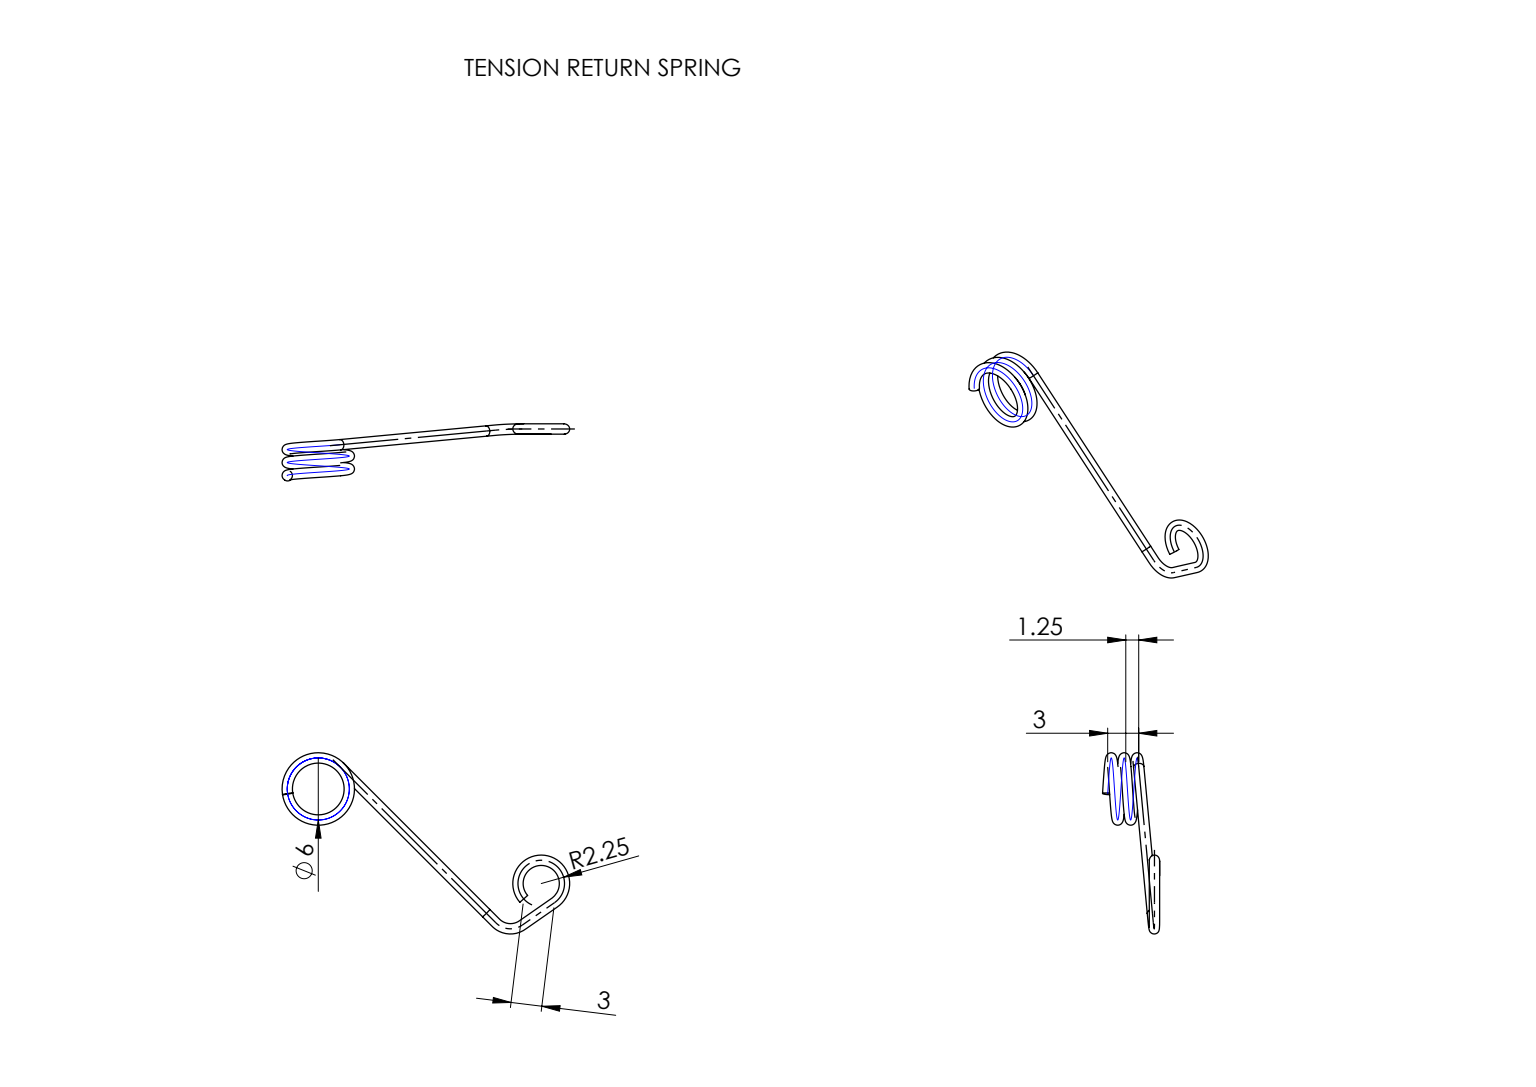
ISO-10303-21;
HEADER;
FILE_DESCRIPTION (('STEP AP214'),
    '1' );
FILE_NAME ('Tension Return Spring.step',
    '2026-10-08T05:45:04',
    ( '' ),
    ( '' ),
    'SwSTEP 2.0',
    'SolidWorks 2026',
    '' );
FILE_SCHEMA (( 'AUTOMOTIVE_DESIGN' ));
ENDSEC;

DATA;
#1=CARTESIAN_POINT ( 'NONE',  ( 16.54959645279592451, 16.98593745313911896, 13.11591282735340336 ) ) ;
#3=CARTESIAN_POINT ( 'NONE',  ( 16.03488360228399046, 17.50065030364834939, 12.16198771834506509 ) ) ;
#5=CARTESIAN_POINT ( 'NONE',  ( 22.63806431670481700, 19.48506897666907989, 12.00579112326951758 ) ) ;
#7=CARTESIAN_POINT ( 'NONE',  ( -2.527408190673963162, 30.96936468028755840, 15.39281658473306358 ) ) ;
#13=ORIENTED_EDGE ( 'NONE', *, *, #10452, .T. ) ;
#17=CARTESIAN_POINT ( 'NONE',  ( 19.95755123817951215, 17.62047157401400810, 12.00579112326941988 ) ) ;
#19=CARTESIAN_POINT ( 'NONE',  ( -2.500000000000005329, 29.80321974748362734, 16.48359592357600789 ) ) ;
#44=CARTESIAN_POINT ( 'NONE',  ( 21.41951502703731691, 22.64547864373410135, 12.00579112326941988 ) ) ;
#48=CARTESIAN_POINT ( 'NONE',  ( 22.57450250028656669, 18.29201386669844709, 10.95195840513859231 ) ) ;
#57=CARTESIAN_POINT ( 'NONE',  ( 3.472591809326047052, 31.51591669395100936, 13.67406658473306535 ) ) ;
#59=CARTESIAN_POINT ( 'NONE',  ( 18.70477062293933557, 21.09978808922912208, 12.94889058896590583 ) ) ;
#60=CARTESIAN_POINT ( 'NONE',  ( 16.65878245872646701, 16.87675144720473952, 12.10347664333366247 ) ) ;
#61=CARTESIAN_POINT ( 'NONE',  ( 17.36588923991300604, 17.58385822839129986, 12.10347664333366247 ) ) ;
#63=CARTESIAN_POINT ( 'NONE',  ( -2.500000000000003997, 29.93383077435482065, 15.47094158473306535 ) ) ;
#71=CARTESIAN_POINT ( 'NONE',  ( 19.29066956973784386, 17.16581860495888634, 12.00630190750973370 ) ) ;
#92=CARTESIAN_POINT ( 'NONE',  ( 20.23853826540680600, 19.71164639310234534, 12.00579112326941988 ) ) ;
#109=CARTESIAN_POINT ( 'NONE',  ( 16.61199375056689931, 16.92354015536430722, 11.10566822806672427 ) ) ;
#116=CARTESIAN_POINT ( 'NONE',  ( -2.521662442312484931, 32.42808502599334730, 12.81469158473306713 ) ) ;
#118=CARTESIAN_POINT ( 'NONE',  ( 22.45649315185626094, 23.58010107951569623, 12.94889058896590583 ) ) ;
#121=CARTESIAN_POINT ( 'NONE',  ( 19.90085419568980640, 16.36478119802090703, 11.95042571680015442 ) ) ;
#122=CARTESIAN_POINT ( 'NONE',  ( 19.29066956973784386, 17.16581860495888634, 12.00630190750973370 ) ) ;
#124=CARTESIAN_POINT ( 'NONE',  ( 2.500000000000008438, 30.00000000000000711, 14.59375000000000178 ) ) ;
#136=CARTESIAN_POINT ( 'NONE',  ( 23.04535143233503192, 19.92821688535955360, 12.00579112326941988 ) ) ;
#140=DIRECTION ( 'NONE',  ( 0.7512361908166118596, 0.6577071706380241967, 0.05536662621717060306 ) ) ;
#145=CARTESIAN_POINT ( 'NONE',  ( 1.101703131577913553, 32.47259180932605460, 17.07593341526694530 ) ) ;
#148=CARTESIAN_POINT ( 'NONE',  ( 2.500000000000007550, 31.03553390593274486, 14.67187500000000178 ) ) ;
#164=CARTESIAN_POINT ( 'NONE',  ( 18.88912242859132107, 19.99746927611068870, 11.95042449705224819 ) ) ;
#173=CARTESIAN_POINT ( 'NONE',  ( -1.515916693951010252, 33.47259180932604750, 13.98656658473306713 ) ) ;
#175=CARTESIAN_POINT ( 'NONE',  ( 22.08651808663882932, 17.88512374315008557, 11.95042449705224819 ) ) ;
#177=CARTESIAN_POINT ( 'NONE',  ( 23.34652552892808330, 18.77429515943753202, 11.95042449705224819 ) ) ;
#196=CARTESIAN_POINT ( 'NONE',  ( -1.814555661125937247, 28.27902175519318817, 16.37280841526694175 ) ) ;
#197=CARTESIAN_POINT ( 'NONE',  ( -2.500000000000005773, 29.99999999999999645, 13.96875000000000355 ) ) ;
#198=UNCERTAINTY_MEASURE_WITH_UNIT (LENGTH_MEASURE( 1.000000000000000082E-05 ), #3270, 'distance_accuracy_value', 'NONE');
#212=CARTESIAN_POINT ( 'NONE',  ( 24.35722724902042202, 20.98982846826517346, 11.95042449705185739 ) ) ;
#213=CARTESIAN_POINT ( 'NONE',  ( 3.500000000000007550, 28.55025253169416644, 15.76562500000000178 ) ) ;
#220=CARTESIAN_POINT ( 'NONE',  ( -0.06616922564517661864, 33.50000000000000000, 12.65844158473306535 ) ) ;
#223=CARTESIAN_POINT ( 'NONE',  ( 24.37916169550391032, 20.40431285142311424, 12.94889058896590761 ) ) ;
#226=CARTESIAN_POINT ( 'NONE',  ( 18.76105380172462844, 21.09515122317004909, 11.95042449705224819 ) ) ;
#228=FACE_OUTER_BOUND ( 'NONE', #3011, .T. ) ;
#235=CARTESIAN_POINT ( 'NONE',  ( 16.74199038346592872, 18.20775708483950694, 12.16198771834549497 ) ) ;
#244=CARTESIAN_POINT ( 'NONE',  ( 1.449747468305833120, 33.50000000000000000, 16.07812500000000355 ) ) ;
#249=CARTESIAN_POINT ( 'NONE',  ( -1.767766952966370209, 28.23223304703362402, 15.37500000000000355 ) ) ;
#250=CARTESIAN_POINT ( 'NONE',  ( -2.500000000000005773, 29.99999999999999645, 16.46875000000000355 ) ) ;
#271=CARTESIAN_POINT ( 'NONE',  ( 23.84774077504003031, 19.42364242282459230, 10.95195840513859231 ) ) ;
#272=CARTESIAN_POINT ( 'NONE',  ( 2.474873734152918558, 32.47487373415292211, 16.00000000000000355 ) ) ;
#279=CARTESIAN_POINT ( 'NONE',  ( -1.814555661125939912, 31.72097824480680117, 15.31469158473306713 ) ) ;
#283=CARTESIAN_POINT ( 'NONE',  ( 23.89484671925281845, 19.39402032390267649, 11.95042449705224819 ) ) ;
#285=CARTESIAN_POINT ( 'NONE',  ( 22.06757164964230711, 19.02077357123424406, 13.00425721518307576 ) ) ;
#300=CARTESIAN_POINT ( 'NONE',  ( -1.515916693951006478, 26.52740819067394895, 16.45093341526693820 ) ) ;
#306=CARTESIAN_POINT ( 'NONE',  ( -2.500000000000007550, 30.06616922564517580, 14.96655841526694175 ) ) ;
#308=AXIS2_PLACEMENT_3D ( 'NONE', #6956, #4296, #9565 ) ;
#310=CARTESIAN_POINT ( 'NONE',  ( 19.29066956973784386, 17.16581860495888634, 12.00630190750973370 ) ) ;
#327=CARTESIAN_POINT ( 'NONE',  ( 19.66613420429507997, 17.48520406133187066, 11.00732503135576401 ) ) ;
#333=CARTESIAN_POINT ( 'NONE',  ( -2.500000000000007550, 31.03553390593274486, 13.89062500000000355 ) ) ;
#335=CARTESIAN_POINT ( 'NONE',  ( 24.30080945327229003, 20.98731269034403368, 10.95195840513820151 ) ) ;
#337=CARTESIAN_POINT ( 'NONE',  ( 19.48730207459019326, 19.05393922246431870, 11.95042449705224996 ) ) ;
#338=CARTESIAN_POINT ( 'NONE',  ( 16.95349311633468403, 16.58206632678699677, 13.07803561935715742 ) ) ;
#343=ORIENTED_EDGE ( 'NONE', *, *, #9950, .F. ) ;
#351=CARTESIAN_POINT ( 'NONE',  ( -2.521662442312484931, 32.42808502599334730, 12.81469158473306713 ) ) ;
#354=CARTESIAN_POINT ( 'NONE',  ( 2.472591809326055046, 28.89829686842209355, 16.76343341526694175 ) ) ;
#375=CARTESIAN_POINT ( 'NONE',  ( 22.78377297911024257, 19.69285065907503807, 11.00732503135576401 ) ) ;
#382=CARTESIAN_POINT ( 'NONE',  ( -2.500000000000004441, 28.96446609406725159, 14.04687500000000355 ) ) ;
#384=CARTESIAN_POINT ( 'NONE',  ( 16.45601903647678910, 17.07951486945825792, 11.12029599681952519 ) ) ;
#387=CARTESIAN_POINT ( 'NONE',  ( 18.14679736200770677, 17.01284808935846371, 13.04404649446423115 ) ) ;
#389=AXIS2_PLACEMENT_3D ( 'NONE', #8545, #5873, #9257 ) ;
#394=CARTESIAN_POINT ( 'NONE',  ( 23.17052989764754756, 21.62756661655841839, 12.00579112326981246 ) ) ;
#402=CARTESIAN_POINT ( 'NONE',  ( -0.06616922564517119243, 26.49999999999999289, 16.52905841526693820 ) ) ;
#406=CARTESIAN_POINT ( 'NONE',  ( -3.472591809326048384, 31.51591669395100936, 14.88843341526694353 ) ) ;
#407=CARTESIAN_POINT ( 'NONE',  ( -1.515916693951006478, 26.52740819067394895, 15.20093341526694353 ) ) ;
#424=CIRCLE ( 'NONE', #2569, 0.5000000000000013323 ) ;
#425=CARTESIAN_POINT ( 'NONE',  ( 23.19605965318632457, 18.72439211931539660, 10.95195840513869179 ) ) ;
#434=CARTESIAN_POINT ( 'NONE',  ( -0.06616922564517727090, 32.50000000000000711, 15.15844158473306535 ) ) ;
#437=CARTESIAN_POINT ( 'NONE',  ( 21.34610222965416071, 23.60463303817794412, 10.95195840513859231 ) ) ;
#443=CARTESIAN_POINT ( 'NONE',  ( 19.16668011427331919, 17.04844365417888596, 13.00677669558776550 ) ) ;
#451=CARTESIAN_POINT ( 'NONE',  ( 21.51635413324704160, 18.70478684647606826, 12.00579112326941988 ) ) ;
#458=CARTESIAN_POINT ( 'NONE',  ( -3.500000000000003553, 31.44974746830583356, 16.39062500000000355 ) ) ;
#464=CARTESIAN_POINT ( 'NONE',  ( -0.06616922564517033201, 27.49999999999998934, 15.27905841526694175 ) ) ;
#481=( BOUNDED_CURVE ( )  B_SPLINE_CURVE ( 3, ( #678, #7459, #10848, #6612 ),
 .UNSPECIFIED., .F., .F. ) 
 B_SPLINE_CURVE_WITH_KNOTS ( ( 4, 4 ),
 ( 0.001563228649568143037, 0.003126104531729810565 ),
 .UNSPECIFIED. ) 
 CURVE ( )  GEOMETRIC_REPRESENTATION_ITEM ( )  RATIONAL_B_SPLINE_CURVE ( ( 1.000000000000000888, 0.3333333333333335369, 0.3333333333333327042, 1.000000000000000000 ) ) 
 REPRESENTATION_ITEM ( '' )  );
#484=AXIS2_PLACEMENT_3D ( 'NONE', #7051, #937, #5776 ) ;
#485=CARTESIAN_POINT ( 'NONE',  ( 21.34610222965416071, 23.60463303817794412, 10.95195840513859231 ) ) ;
#497=CARTESIAN_POINT ( 'NONE',  ( 16.37803167940877458, 17.15750222652490820, 11.12760988119559258 ) ) ;
#502=CARTESIAN_POINT ( 'NONE',  ( 22.73223279825284848, 19.49146071982302075, 13.00425721518307753 ) ) ;
#508=CARTESIAN_POINT ( 'NONE',  ( 21.90605485701305000, 18.97586566459109392, 12.00579112326941988 ) ) ;
#513=CARTESIAN_POINT ( 'NONE',  ( 3.527408190673962274, 28.61642175733934934, 14.76781658473306535 ) ) ;
#518=CARTESIAN_POINT ( 'NONE',  ( -3.500000000000005329, 30.06616922564516869, 16.21655841526694175 ) ) ;
#534=CARTESIAN_POINT ( 'NONE',  ( 22.29575558078030895, 19.24694448270711788, 12.00579112326941988 ) ) ;
#540=CARTESIAN_POINT ( 'NONE',  ( 1.767766952966377314, 28.23223304703363112, 15.68750000000000355 ) ) ;
#544=CARTESIAN_POINT ( 'NONE',  ( 20.23629815768686768, 16.66554095800588797, 10.95195840513859231 ) ) ;
#546=CARTESIAN_POINT ( 'NONE',  ( 22.63773560303409127, 18.20111046790825782, 12.94889058896590583 ) ) ;
#554=CARTESIAN_POINT ( 'NONE',  ( 20.47715220320264962, 17.98190999816754498, 12.00579112326941988 ) ) ;
#561=CARTESIAN_POINT ( 'NONE',  ( 1.814555661125942132, 28.27902175519319883, 13.43969158473306713 ) ) ;
#567=CARTESIAN_POINT ( 'NONE',  ( -2.479565268636987785, 29.67421718125152452, 17.49702953738633937 ) ) ;
#571=CARTESIAN_POINT ( 'NONE',  ( -1.035533905932736420, 27.49999999999998934, 14.20312500000000355 ) ) ;
#578=CARTESIAN_POINT ( 'NONE',  ( -2.474873734152920335, 32.47487373415291501, 15.06250000000000355 ) ) ;
#585=CARTESIAN_POINT ( 'NONE',  ( 19.84380896203909828, 21.37294244821887546, 12.00579112326902731 ) ) ;
#595=CARTESIAN_POINT ( 'NONE',  ( 4.553649124439118623E-15, 27.49999999999999289, 15.53125000000000355 ) ) ;
#597=CARTESIAN_POINT ( 'NONE',  ( 17.60432978939287452, 17.35624782240900288, 11.07951759511215606 ) ) ;
#598=PRESENTATION_STYLE_ASSIGNMENT (( #4897 ) ) ;
#602=CARTESIAN_POINT ( 'NONE',  ( 19.75845051886964043, 23.09045650430892849, 12.94889058896590583 ) ) ;
#610=CARTESIAN_POINT ( 'NONE',  ( -1.515916693951006478, 26.52740819067394895, 16.45093341526693820 ) ) ;
#613=CARTESIAN_POINT ( 'NONE',  ( 19.55162244606592381, 17.33808635661342024, 12.00579012602852735 ) ) ;
#619=CARTESIAN_POINT ( 'NONE',  ( -3.472591809326043499, 28.48408330604899064, 14.29906658473306358 ) ) ;
#627=CARTESIAN_POINT ( 'NONE',  ( -3.500000000000005329, 30.06616922564516869, 14.96655841526694175 ) ) ;
#640=CARTESIAN_POINT ( 'NONE',  ( 1.449747468305836673, 26.49999999999999289, 14.35937500000000533 ) ) ;
#644=CARTESIAN_POINT ( 'NONE',  ( 19.35452611835372849, 17.20101589911864437, 12.00579185514580338 ) ) ;
#657=CARTESIAN_POINT ( 'NONE',  ( 20.21677217982034946, 21.95921345637081501, 11.00732503135595941 ) ) ;
#661=CARTESIAN_POINT ( 'NONE',  ( 22.11813463801259161, 17.83967204375498383, 12.94889058896590583 ) ) ;
#669=CARTESIAN_POINT ( 'NONE',  ( -1.720978244806810498, 31.81455566112594013, 17.31030841526694175 ) ) ;
#671=CARTESIAN_POINT ( 'NONE',  ( 19.95752144772427528, 19.94857296576799754, 13.00425721518131184 ) ) ;
#677=CARTESIAN_POINT ( 'NONE',  ( -3.500000000000001332, 29.93383077435482065, 12.97094158473306358 ) ) ;
#678=CARTESIAN_POINT ( 'NONE',  ( 15.87890888817147150, 17.65662501776163040, 12.17661548709639341 ) ) ;
#692=CARTESIAN_POINT ( 'NONE',  ( -1.767766952966375094, 31.76776695296636888, 13.81250000000000355 ) ) ;
#696=CARTESIAN_POINT ( 'NONE',  ( 17.79249663040192431, 17.21067465782413919, 12.06642298039558980 ) ) ;
#704=CARTESIAN_POINT ( 'NONE',  ( -1.035533905932736420, 27.49999999999998934, 15.45312500000000178 ) ) ;
#706=CARTESIAN_POINT ( 'NONE',  ( 17.20991452582289583, 17.73983294248524700, 12.11810441208646338 ) ) ;
#710=CARTESIAN_POINT ( 'NONE',  ( 19.07396262421655919, 19.44200532275891291, 12.94889058896472811 ) ) ;
#716=SHAPE_REPRESENTATION ( 'Tension Return Spring', ( #308 ), #3340 ) ;
#717=CARTESIAN_POINT ( 'NONE',  ( 2.521662442312485819, 32.42808502599335441, 14.49780841526694175 ) ) ;
#719=CARTESIAN_POINT ( 'NONE',  ( 24.08125446323534291, 19.61299372598402613, 12.94889058896590761 ) ) ;
#725=CARTESIAN_POINT ( 'NONE',  ( -2.500000000000003997, 29.93383077435482065, 14.22094158473306535 ) ) ;
#733=CARTESIAN_POINT ( 'NONE',  ( 23.17052989764754756, 21.62756661655841839, 12.00579112326981246 ) ) ;
#742=CARTESIAN_POINT ( 'NONE',  ( 1.767766952966377314, 28.23223304703363112, 14.43750000000000178 ) ) ;
#746=CARTESIAN_POINT ( 'NONE',  ( 19.29066956973784386, 17.16581860495888634, 12.00630190750973370 ) ) ;
#757=CARTESIAN_POINT ( 'NONE',  ( 17.65010306112908722, 17.31038946799904465, 12.07741653513508417 ) ) ;
#760=CARTESIAN_POINT ( 'NONE',  ( 18.97799213218983994, 15.95698123192398477, 12.96557279687576525 ) ) ;
#769=CARTESIAN_POINT ( 'NONE',  ( 2.521662442312485819, 32.42808502599335441, 16.99780841526693820 ) ) ;
#773=CARTESIAN_POINT ( 'NONE',  ( 20.12931512496741249, 22.03068688373604900, 13.00425721518366728 ) ) ;
#775=CARTESIAN_POINT ( 'NONE',  ( 22.60611905166032898, 18.24656216730335601, 11.95042449705224819 ) ) ;
#779=CARTESIAN_POINT ( 'NONE',  ( -2.494791681227495950, 29.73705052183845154, 15.48578750830907147 ) ) ;
#789=CARTESIAN_POINT ( 'NONE',  ( 21.51635413324704160, 18.70478684647606826, 12.00579112326941988 ) ) ;
#807=CARTESIAN_POINT ( 'NONE',  ( 19.85760542366876535, 20.31250532737884384, 12.00579112326941988 ) ) ;
#818=CARTESIAN_POINT ( 'NONE',  ( 19.66613420429507997, 17.48520406133187066, 11.00732503135576401 ) ) ;
#824=CARTESIAN_POINT ( 'NONE',  ( 15.36174878203077476, 18.17378512388119915, 11.22291988893967840 ) ) ;
#835=CARTESIAN_POINT ( 'NONE',  ( 1.383578242660657098, 33.52740819067396671, 15.08031658473306891 ) ) ;
#837=CARTESIAN_POINT ( 'NONE',  ( 19.53332707643461319, 16.11782042516817981, 12.95310296989756260 ) ) ;
#839=EDGE_CURVE ( 'NONE', #8937, #5318, #2844, .T. ) ;
#845=CARTESIAN_POINT ( 'NONE',  ( 1.035533905932737975, 32.50000000000000711, 13.57812500000000178 ) ) ;
#856=CARTESIAN_POINT ( 'NONE',  ( 22.69616945897178084, 19.53356342368596898, 12.00579112326941988 ) ) ;
#857=CARTESIAN_POINT ( 'NONE',  ( -1.035533905932736420, 27.49999999999998934, 15.45312500000000178 ) ) ;
#882=CARTESIAN_POINT ( 'NONE',  ( 22.05490153526506703, 17.93057544254518376, 10.95195840513859231 ) ) ;
#883=CARTESIAN_POINT ( 'NONE',  ( -3.456897879362374582, 29.45240795142739998, 16.49922112211940117 ) ) ;
#890=CARTESIAN_POINT ( 'NONE',  ( -3.500000000000003553, 31.44974746830583356, 16.39062500000000355 ) ) ;
#893=CARTESIAN_POINT ( 'NONE',  ( 21.85833415550051484, 17.65895283167741425, 12.94889058896590583 ) ) ;
#896=CARTESIAN_POINT ( 'NONE',  ( 17.59356678224322934, 17.35619608210146581, 12.08212522340233264 ) ) ;
#898=CARTESIAN_POINT ( 'NONE',  ( -1.767766952966370209, 28.23223304703362402, 15.37500000000000355 ) ) ;
#909=CARTESIAN_POINT ( 'NONE',  ( -2.385244779468109755E-15, 32.50000000000000711, 16.15625000000000355 ) ) ;
#937=DIRECTION ( 'NONE',  ( -0.1561119869139967753, 0.9855205127846311530, -0.06616922564517428718 ) ) ;
#939=CARTESIAN_POINT ( 'NONE',  ( 24.09141472773967507, 22.06251279622207306, 11.95042449705264076 ) ) ;
#946=CARTESIAN_POINT ( 'NONE',  ( 0.06616922564517879746, 26.50000000000000000, 13.28344158473306713 ) ) ;
#948=CARTESIAN_POINT ( 'NONE',  ( 21.34179237787287065, 23.66094220255952152, 11.95042449705224819 ) ) ;
#950=CARTESIAN_POINT ( 'NONE',  ( 18.94130700685887447, 16.00034706198404066, 11.96718634320919250 ) ) ;
#951=CARTESIAN_POINT ( 'NONE',  ( 15.88045857259785087, 19.06928889570832197, 12.24278471274156388 ) ) ;
#960=CARTESIAN_POINT ( 'NONE',  ( 18.10462311893278553, 17.05669763433401087, 12.04589798090090902 ) ) ;
#971=EDGE_LOOP ( 'NONE', ( #10177, #7485, #4128, #4625 ) ) ;
#974=CARTESIAN_POINT ( 'NONE',  ( -1.101703131577911776, 27.52740819067395250, 16.45093341526693820 ) ) ;
#994=CARTESIAN_POINT ( 'NONE',  ( 17.22114890795359798, 16.40384437412513208, 11.05348780010051435 ) ) ;
#1002=CARTESIAN_POINT ( 'NONE',  ( 1.449747468305836673, 26.49999999999999289, 15.60937500000000711 ) ) ;
#1004=CARTESIAN_POINT ( 'NONE',  ( 19.79393261808261428, 23.04652112618272852, 11.95042449705224819 ) ) ;
#1006=CARTESIAN_POINT ( 'NONE',  ( 24.35722724902042202, 20.98982846826517346, 11.95042449705185739 ) ) ;
#1007=CARTESIAN_POINT ( 'NONE',  ( 19.35452611835372849, 17.20101589911864437, 12.00579185514580338 ) ) ;
#1009=CARTESIAN_POINT ( 'NONE',  ( -2.500000000000004885, 29.80321974748363090, 16.48359592357600434 ) ) ;
#1011=CARTESIAN_POINT ( 'NONE',  ( -0.06616922564517661864, 33.50000000000000000, 15.15844158473306535 ) ) ;
#1021=CARTESIAN_POINT ( 'NONE',  ( -2.500000000000007550, 31.03553390593274131, 16.39062500000000355 ) ) ;
#1030=CARTESIAN_POINT ( 'NONE',  ( -2.500000000000005773, 29.99999999999999645, 15.21875000000000355 ) ) ;
#1032=CARTESIAN_POINT ( 'NONE',  ( 1.767766952966372429, 31.76776695296637598, 14.75000000000000355 ) ) ;
#1048=CARTESIAN_POINT ( 'NONE',  ( 19.86895450806392560, 16.41003605044161162, 10.95195963068177392 ) ) ;
#1049=CARTESIAN_POINT ( 'NONE',  ( -2.474873734152920335, 32.47487373415291501, 16.31250000000000355 ) ) ;
#1051=ADVANCED_FACE ( 'NONE', ( #228 ), #4624, .T. ) ;
#1056=CARTESIAN_POINT ( 'NONE',  ( -2.521662442312484931, 32.42808502599334730, 14.06469158473306358 ) ) ;
#1058=CARTESIAN_POINT ( 'NONE',  ( 23.34652552892808330, 18.77429515943753202, 11.95042449705224819 ) ) ;
#1060=CARTESIAN_POINT ( 'NONE',  ( 23.64018263364375017, 19.06693133664117212, 11.95042449705224819 ) ) ;
#1061=CARTESIAN_POINT ( 'NONE',  ( 22.45328846257175925, 22.40877220821986171, 12.00579112326941988 ) ) ;
#1077=CARTESIAN_POINT ( 'NONE',  ( -3.472591809326048384, 31.51591669395100936, 17.38843341526693820 ) ) ;
#1082=CARTESIAN_POINT ( 'NONE',  ( 2.500000000000010214, 28.96446609406726225, 14.51562500000000355 ) ) ;
#1102=CARTESIAN_POINT ( 'NONE',  ( 21.87443830563928415, 19.02131736398618855, 11.00732503135576401 ) ) ;
#1110=CARTESIAN_POINT ( 'NONE',  ( -2.500000000000003997, 29.93383077435482065, 12.97094158473306358 ) ) ;
#1113=CARTESIAN_POINT ( 'NONE',  ( 20.26791470906062997, 16.62008925861079334, 11.95042449705224819 ) ) ;
#1116=CARTESIAN_POINT ( 'NONE',  ( 19.79393261808261428, 23.04652112618272852, 11.95042449705224819 ) ) ;
#1118=CARTESIAN_POINT ( 'NONE',  ( 19.05040816462259556, 17.06282649731835122, 12.00984920396035172 ) ) ;
#1124=CARTESIAN_POINT ( 'NONE',  ( 17.45361707773674809, 17.49611573659335662, 12.09524845743996657 ) ) ;
#1131=CARTESIAN_POINT ( 'NONE',  ( -1.734723475976807094E-15, 33.50000000000000000, 16.15625000000000355 ) ) ;
#1136=CARTESIAN_POINT ( 'NONE',  ( -2.385244779468109755E-15, 32.50000000000000711, 14.90625000000000355 ) ) ;
#1137=CARTESIAN_POINT ( 'NONE',  ( -3.456897879362374582, 29.45240795142739998, 16.49922112211940117 ) ) ;
#1159=CARTESIAN_POINT ( 'NONE',  ( 24.30080945327229003, 20.98731269034403368, 10.95195840513820151 ) ) ;
#1166=CARTESIAN_POINT ( 'NONE',  ( 2.472591809326049272, 31.10170313157791711, 14.92406658473306713 ) ) ;
#1169=CARTESIAN_POINT ( 'NONE',  ( 24.41364504476855402, 20.99234424618630257, 12.94889058896551326 ) ) ;
#1170=APPLICATION_CONTEXT ( 'automotive_design' ) ;
#1172=CARTESIAN_POINT ( 'NONE',  ( 17.41267794807257374, 17.53706952023173216, 13.10128505860060066 ) ) ;
#1175=SURFACE_SIDE_STYLE ('',( #8791 ) ) ;
#1182=CARTESIAN_POINT ( 'NONE',  ( 17.20991452582289583, 17.73983294248524700, 12.11810441208646338 ) ) ;
#1190=CARTESIAN_POINT ( 'NONE',  ( 2.474873734152922111, 27.52512626584708144, 15.68750000000000355 ) ) ;
#1194=ADVANCED_FACE ( 'NONE', ( #10156 ), #7826, .T. ) ;
#1195=CARTESIAN_POINT ( 'NONE',  ( 0.06616922564517249694, 32.50000000000000711, 15.90405841526694175 ) ) ;
#1198=CARTESIAN_POINT ( 'NONE',  ( -2.500000000000005773, 29.99999999999999645, 15.21875000000000355 ) ) ;
#1222=CARTESIAN_POINT ( 'NONE',  ( 22.00433854689477897, 19.11167697002443333, 11.00732503135576401 ) ) ;
#1229=CARTESIAN_POINT ( 'NONE',  ( 1.101703131577918438, 27.52740819067395606, 13.36156658473306535 ) ) ;
#1230=ORIENTED_EDGE ( 'NONE', *, *, #839, .F. ) ;
#1231=CARTESIAN_POINT ( 'NONE',  ( 18.81733698050991777, 21.09051435711097966, 10.95195840513859231 ) ) ;
#1233=CARTESIAN_POINT ( 'NONE',  ( 22.98142095123195716, 18.50759888342988546, 11.95042449705211141 ) ) ;
#1234=CARTESIAN_POINT ( 'NONE',  ( 19.08509339279509831, 17.01892842213374735, 13.00828316275149099 ) ) ;
#1238=B_SPLINE_CURVE_WITH_KNOTS ( 'NONE', 3,
 ( #9810, #2255, #5649, #4814, #1472, #4083, #4023, #7411, #10804, #9128, #10026, #2415, #5802, #6798, #7585, #5092, #7642, #71, #4980, #6077, #10307, #17, #9361, #4257, #3418, #10253, #789, #10193, #1759, #1694, #8472, #2590, #856, #3536, #2702, #136, #5971, #5913, #10975, #733, #9296, #3364, #6918, #8579, #6743, #1581, #5150, #2475, #4196, #3306, #8354, #10139 ),
 .UNSPECIFIED., .F., .F.,
 ( 4, 2, 2, 2, 2, 2, 2, 2, 2, 2, 2, 2, 2, 2, 2, 2, 2, 2, 2, 2, 2, 2, 2, 2, 2, 4 ),
 ( 0.05059550242215297977, 0.08415034466753114339, 0.1009277657902202252, 0.1177051869129092931, 0.1353321994545625961, 0.1529592119962158714, 0.1882132370795224774, 0.2234672621628290834, 0.2410942747044824142, 0.2587212872461356894, 0.2827395206008344042, 0.3067577539555331190, 0.3547942206649305485, 0.4028306873743279781, 0.4268489207290267484, 0.4508671540837254077, 0.4680275555186089731, 0.4851879569534925385, 0.5195087598232597248, 0.5881503655627940974, 0.6567919713023284700, 0.7254335770418627316, 0.7940751827813969932, 0.8627167885209312548, 0.9313583942604657384, 1.000000000000000000 ),
 .UNSPECIFIED. ) ;
#1243=CARTESIAN_POINT ( 'NONE',  ( 15.92724728075741680, 19.02250018754875072, 13.24059312800850030 ) ) ;
#1252=CARTESIAN_POINT ( 'NONE',  ( -2.474873734152920335, 32.47487373415291501, 13.81250000000000355 ) ) ;
#1257=CARTESIAN_POINT ( 'NONE',  ( -1.383578242660661983, 33.52740819067396671, 15.98218341526694175 ) ) ;
#1258=CARTESIAN_POINT ( 'NONE',  ( 1.515916693951008254, 33.47259180932604750, 15.82593341526694353 ) ) ;
#1259=CARTESIAN_POINT ( 'NONE',  ( 22.45328846257175925, 22.40877220821986171, 12.00579112326941988 ) ) ;
#1278=CARTESIAN_POINT ( 'NONE',  ( 19.52895938645546536, 19.09041019265748673, 10.95195840513859586 ) ) ;
#1284=CARTESIAN_POINT ( 'NONE',  ( 2.472591809326049272, 31.10170313157791711, 13.67406658473306535 ) ) ;
#1286=CARTESIAN_POINT ( 'NONE',  ( 15.12656308325174415, 18.40897082268132934, 11.24497629747462568 ) ) ;
#1291=CARTESIAN_POINT ( 'NONE',  ( 17.50063742165245984, 17.44909550871243198, 13.09303515564029397 ) ) ;
#1297=CARTESIAN_POINT ( 'NONE',  ( 20.00651627240589647, 19.97666299463432438, 12.00579112326824216 ) ) ;
#1304=CARTESIAN_POINT ( 'NONE',  ( -1.383578242660661983, 33.52740819067396671, 17.23218341526694530 ) ) ;
#1308=CARTESIAN_POINT ( 'NONE',  ( 0.9693646802875698354, 27.47259180932603684, 16.60718341526694175 ) ) ;
#1328=CARTESIAN_POINT ( 'NONE',  ( 23.59820535295391508, 19.10314065948846718, 10.95195840513859231 ) ) ;
#1335=CARTESIAN_POINT ( 'NONE',  ( -2.500000000000007550, 31.03553390593274486, 15.14062500000000355 ) ) ;
#1339=CARTESIAN_POINT ( 'NONE',  ( 16.69520167530635746, 18.25454579299907465, 11.16417930307855677 ) ) ;
#1344=CARTESIAN_POINT ( 'NONE',  ( 17.25670323398246353, 17.69304423432567930, 13.11591282735340336 ) ) ;
#1353=CARTESIAN_POINT ( 'NONE',  ( 22.03595509826854126, 19.06622527062933870, 12.00579112326941988 ) ) ;
#1360=CARTESIAN_POINT ( 'NONE',  ( -3.472591809326043499, 28.48408330604899064, 13.04906658473306891 ) ) ;
#1365=CARTESIAN_POINT ( 'NONE',  ( -1.383578242660661983, 33.52740819067396671, 15.98218341526694175 ) ) ;
#1369=CARTESIAN_POINT ( 'NONE',  ( -1.035533905932742860, 32.50000000000000000, 13.73437500000000888 ) ) ;
#1374=ORIENTED_EDGE ( 'NONE', *, *, #8914, .F. ) ;
#1385=CARTESIAN_POINT ( 'NONE',  ( 18.79784185921769790, 16.99560944861731215, 12.01584860934582366 ) ) ;
#1399=CARTESIAN_POINT ( 'NONE',  ( 19.42818427286271898, 22.60367925258928068, 10.95195840513898489 ) ) ;
#1401=CARTESIAN_POINT ( 'NONE',  ( 23.09245737654782360, 19.89859478643763069, 13.00425721518307753 ) ) ;
#1409=CARTESIAN_POINT ( 'NONE',  ( 19.16668011427331919, 17.04844365417888596, 13.00677669558776550 ) ) ;
#1414=CARTESIAN_POINT ( 'NONE',  ( -3.446545381698513655, 29.38705359262400663, 15.50141270685246830 ) ) ;
#1420=CARTESIAN_POINT ( 'NONE',  ( -2.527408190673963162, 29.03063531971243094, 16.29468341526694530 ) ) ;
#1429=CARTESIAN_POINT ( 'NONE',  ( -3.500000000000003109, 29.99999999999999645, 13.96875000000000355 ) ) ;
#1434=CARTESIAN_POINT ( 'NONE',  ( 16.11564427137601285, 18.83410319690818824, 12.22072830420661660 ) ) ;
#1442=CARTESIAN_POINT ( 'NONE',  ( -2.500000000000007550, 31.03553390593274486, 16.39062500000000355 ) ) ;
#1446=CARTESIAN_POINT ( 'NONE',  ( 21.07346791105437589, 22.52558620363005915, 11.00732503135576401 ) ) ;
#1450=CARTESIAN_POINT ( 'NONE',  ( 23.83741617020655212, 22.59052263540754524, 12.94889058896590583 ) ) ;
#1455=CARTESIAN_POINT ( 'NONE',  ( 2.428085025993357071, 27.47833755768751374, 15.43530841526694175 ) ) ;
#1457=CARTESIAN_POINT ( 'NONE',  ( 20.76856923708738734, 18.11717751085002703, 13.00425721518307576 ) ) ;
#1465=CARTESIAN_POINT ( 'NONE',  ( 2.527408190673965382, 29.03063531971243449, 13.51781658473306713 ) ) ;
#1470=CARTESIAN_POINT ( 'NONE',  ( -0.06616922564517033201, 27.49999999999998934, 16.52905841526693820 ) ) ;
#1472=CARTESIAN_POINT ( 'NONE',  ( 17.20991452582289583, 17.73983294248524700, 12.11810441208646338 ) ) ;
#1479=CARTESIAN_POINT ( 'NONE',  ( -1.449747468305830678, 26.49999999999999289, 15.45312500000000178 ) ) ;
#1483=CARTESIAN_POINT ( 'NONE',  ( 19.55162244606592381, 17.33808635661342024, 12.00579012602852735 ) ) ;
#1494=CARTESIAN_POINT ( 'NONE',  ( 16.74199038346592872, 18.20775708483950694, 12.16198771834549497 ) ) ;
#1500=CARTESIAN_POINT ( 'NONE',  ( 23.58716357997163016, 18.92604383881832675, 12.94889058896590583 ) ) ;
#1506=CARTESIAN_POINT ( 'NONE',  ( -0.06616922564517119243, 26.49999999999999289, 15.27905841526694175 ) ) ;
#1509=CARTESIAN_POINT ( 'NONE',  ( 16.23764702455707720, 17.29788688137487185, 13.14516836485838169 ) ) ;
#1515=CARTESIAN_POINT ( 'NONE',  ( 1.720978244806805169, 31.81455566112594013, 12.50219158473306358 ) ) ;
#1535=CARTESIAN_POINT ( 'NONE',  ( 3.903127820947815962E-15, 26.49999999999999289, 15.53125000000000355 ) ) ;
#1540=CARTESIAN_POINT ( 'NONE',  ( 17.20991452582289583, 17.73983294248524700, 12.11810441208646338 ) ) ;
#1553=CARTESIAN_POINT ( 'NONE',  ( 22.41005638895160601, 19.39388128063383476, 11.00732503135576401 ) ) ;
#1557=CARTESIAN_POINT ( 'NONE',  ( 24.37916169550391032, 20.40431285142311424, 12.94889058896590761 ) ) ;
#1565=CARTESIAN_POINT ( 'NONE',  ( -0.06616922564517119243, 26.49999999999999289, 16.52905841526693820 ) ) ;
#1567=CARTESIAN_POINT ( 'NONE',  ( 23.18216631463591781, 20.05868775325893338, 13.00425721518307753 ) ) ;
#1573=CARTESIAN_POINT ( 'NONE',  ( -0.06616922564517727090, 32.50000000000000711, 13.90844158473306713 ) ) ;
#1581=CARTESIAN_POINT ( 'NONE',  ( 20.43380676890320657, 22.25420293214091316, 12.00579112326941988 ) ) ;
#1591=CARTESIAN_POINT ( 'NONE',  ( -2.500000000000004441, 28.96446609406725159, 14.04687500000000355 ) ) ;
#1596=CARTESIAN_POINT ( 'NONE',  ( 18.10462311893278553, 17.05669763433401087, 12.04589798090090902 ) ) ;
#1606=CARTESIAN_POINT ( 'NONE',  ( -2.500000000000004885, 29.80321974748363090, 16.48359592357600434 ) ) ;
#1608=CARTESIAN_POINT ( 'NONE',  ( 19.25788680476432546, 17.21053220311310739, 11.00783986014182148 ) ) ;
#1612=CARTESIAN_POINT ( 'NONE',  ( 24.41364504476855402, 20.99234424618630257, 12.94889058896551326 ) ) ;
#1620=CARTESIAN_POINT ( 'NONE',  ( -1.383578242660661983, 33.52740819067396671, 17.23218341526694530 ) ) ;
#1623=CARTESIAN_POINT ( 'NONE',  ( 22.50783536177859645, 18.11075086187001659, 12.94889058896590583 ) ) ;
#1625=VECTOR ( 'NONE', #10324, 999.9999999999998863 ) ;
#1626=CARTESIAN_POINT ( 'NONE',  ( 22.47621881040483771, 18.15620256126511478, 11.95042449705224819 ) ) ;
#1630=CARTESIAN_POINT ( 'NONE',  ( 1.814555661125942132, 28.27902175519319883, 14.68969158473306535 ) ) ;
#1663=CARTESIAN_POINT ( 'NONE',  ( 22.00433854689477897, 19.11167697002443333, 11.00732503135576401 ) ) ;
#1667=CARTESIAN_POINT ( 'NONE',  ( 22.43871220627207563, 23.52649944903870249, 11.95042449705224819 ) ) ;
#1674=CARTESIAN_POINT ( 'NONE',  ( 3.527408190673962274, 28.61642175733934934, 14.76781658473306535 ) ) ;
#1676=CARTESIAN_POINT ( 'NONE',  ( 23.01143949934618504, 18.46103507366711227, 12.94889058896576906 ) ) ;
#1683=CARTESIAN_POINT ( 'NONE',  ( 2.472591809326049272, 31.10170313157791711, 14.92406658473306713 ) ) ;
#1689=ADVANCED_FACE ( 'NONE', ( #4201 ), #10919, .T. ) ;
#1694=CARTESIAN_POINT ( 'NONE',  ( 22.29575558078030895, 19.24694448270711788, 12.00579112326941988 ) ) ;
#1696=CARTESIAN_POINT ( 'NONE',  ( 2.500000000000008438, 30.00000000000000711, 15.84375000000000355 ) ) ;
#1720=CARTESIAN_POINT ( 'NONE',  ( 21.25655365073496839, 18.52406763439849513, 12.00579112326941988 ) ) ;
#1726=CARTESIAN_POINT ( 'NONE',  ( 21.01569960522067504, 17.20769859423666048, 10.95195840513859231 ) ) ;
#1737=CARTESIAN_POINT ( 'NONE',  ( -3.446545381698513655, 29.38705359262400663, 15.50141270685246830 ) ) ;
#1739=CARTESIAN_POINT ( 'NONE',  ( 20.19688095354152324, 19.67517542290917731, 13.00425721518307753 ) ) ;
#1744=CARTESIAN_POINT ( 'NONE',  ( 21.05771646464872404, 22.57981893131178452, 12.00579112326941988 ) ) ;
#1746=CARTESIAN_POINT ( 'NONE',  ( -1.767766952966375094, 31.76776695296636888, 16.31250000000000355 ) ) ;
#1759=CARTESIAN_POINT ( 'NONE',  ( 22.03595509826854126, 19.06622527062933870, 12.00579112326941988 ) ) ;
#1760=CARTESIAN_POINT ( 'NONE',  ( 2.500000000000008438, 30.00000000000000711, 14.59375000000000178 ) ) ;
#1781=CARTESIAN_POINT ( 'NONE',  ( 20.08745147943499987, 17.71083118005251933, 12.00579112326941988 ) ) ;
#1786=CARTESIAN_POINT ( 'NONE',  ( 19.38445574543743177, 22.63941596627307362, 11.95042449705263898 ) ) ;
#1787=CARTESIAN_POINT ( 'NONE',  ( 3.500000000000005329, 30.00000000000000000, 15.84375000000000355 ) ) ;
#1793=CARTESIAN_POINT ( 'NONE',  ( -3.472591809326043499, 28.48408330604899064, 13.04906658473306891 ) ) ;
#1795=CARTESIAN_POINT ( 'NONE',  ( 16.72700999897183038, 16.80849948458634557, 12.09707671258119888 ) ) ;
#1798=CARTESIAN_POINT ( 'NONE',  ( 17.78598590678423719, 16.10215687441832699, 12.01726674494117653 ) ) ;
#1799=CARTESIAN_POINT ( 'NONE',  ( 20.23853826540680600, 19.71164639310234534, 12.00579112326941988 ) ) ;
#1801=CARTESIAN_POINT ( 'NONE',  ( -2.469212770973128190, 29.60886282244813117, 16.49922112211940117 ) ) ;
#1806=ORIENTED_EDGE ( 'NONE', *, *, #6807, .F. ) ;
#1818=CARTESIAN_POINT ( 'NONE',  ( -1.767766952966375094, 31.76776695296636888, 16.31250000000000355 ) ) ;
#1836=CARTESIAN_POINT ( 'NONE',  ( 20.26791470906062997, 16.62008925861079334, 11.95042449705224819 ) ) ;
#1843=CARTESIAN_POINT ( 'NONE',  ( 3.500000000000003997, 30.06616922564517580, 14.84594158473306713 ) ) ;
#1845=CARTESIAN_POINT ( 'NONE',  ( 19.76265562249496099, 16.28401831655332543, 11.95127577209155234 ) ) ;
#1850=CARTESIAN_POINT ( 'NONE',  ( 1.035533905932743970, 27.49999999999999289, 15.60937500000000711 ) ) ;
#1860=CARTESIAN_POINT ( 'NONE',  ( -2.469212770973128190, 29.60886282244813827, 16.49922112211940117 ) ) ;
#1871=CARTESIAN_POINT ( 'NONE',  ( 2.500000000000009770, 29.93383077435482420, 16.84155841526694175 ) ) ;
#1897=CARTESIAN_POINT ( 'NONE',  ( 18.60991190964745456, 16.01828113007465504, 10.97873183052796620 ) ) ;
#1906=CARTESIAN_POINT ( 'NONE',  ( -1.734723475976807094E-15, 33.50000000000000000, 16.15625000000000355 ) ) ;
#1908=CARTESIAN_POINT ( 'NONE',  ( 18.07012887690021330, 16.02595819568259827, 12.00212024154935975 ) ) ;
#1931=ORIENTED_EDGE ( 'NONE', *, *, #7024, .F. ) ;
#1934=CARTESIAN_POINT ( 'NONE',  ( 2.500000000000010214, 28.96446609406726225, 15.76562500000000178 ) ) ;
#1955=CARTESIAN_POINT ( 'NONE',  ( 16.69520167530635746, 18.25454579299907465, 11.16417930307855677 ) ) ;
#1962=CARTESIAN_POINT ( 'NONE',  ( -0.9693646802875608426, 27.47259180932603684, 14.45531658473306535 ) ) ;
#1964=CARTESIAN_POINT ( 'NONE',  ( 16.90694777372845437, 16.62861179130368683, 12.08020438729360180 ) ) ;
#1966=CARTESIAN_POINT ( 'NONE',  ( 19.95755123817951215, 17.62047157401400810, 12.00579112326941988 ) ) ;
#1979=CARTESIAN_POINT ( 'NONE',  ( -3.500000000000005329, 30.06616922564516869, 17.46655841526694175 ) ) ;
#1984=CARTESIAN_POINT ( 'NONE',  ( -2.469212770973128190, 29.60886282244813117, 16.49922112211940117 ) ) ;
#1985=CARTESIAN_POINT ( 'NONE',  ( 1.767766952966377314, 28.23223304703363112, 14.43750000000000178 ) ) ;
#2000=CARTESIAN_POINT ( 'NONE',  ( 23.26254143866440671, 20.58647472722595850, 11.00732503135576401 ) ) ;
#2002=CARTESIAN_POINT ( 'NONE',  ( -3.500000000000002665, 29.72450764647708255, 16.48359592357600789 ) ) ;
#2010=CARTESIAN_POINT ( 'NONE',  ( -1.814555661125939912, 31.72097824480680117, 14.06469158473306358 ) ) ;
#2012=CARTESIAN_POINT ( 'NONE',  ( 15.40853749019034069, 18.12699641572163145, 12.22072830420661660 ) ) ;
#2013=CARTESIAN_POINT ( 'NONE',  ( 18.86745781575159242, 21.66267592685425569, 11.95042449705185561 ) ) ;
#2014=CARTESIAN_POINT ( 'NONE',  ( 21.93767140838681584, 18.93041396519599928, 13.00425721518307576 ) ) ;
#2028=CARTESIAN_POINT ( 'NONE',  ( 3.500000000000005773, 31.44974746830583356, 14.67187500000000178 ) ) ;
#2034=CARTESIAN_POINT ( 'NONE',  ( 1.767766952966372429, 31.76776695296637598, 16.00000000000000355 ) ) ;
#2037=CARTESIAN_POINT ( 'NONE',  ( 21.51635413324704160, 18.70478684647606826, 12.00579112326941988 ) ) ;
#2057=CARTESIAN_POINT ( 'NONE',  ( 19.42818427286271898, 22.60367925258928068, 10.95195840513898489 ) ) ;
#2064=CARTESIAN_POINT ( 'NONE',  ( -2.458860273309268152, 29.54350846364475203, 15.50141270685246830 ) ) ;
#2067=CARTESIAN_POINT ( 'NONE',  ( 18.88912242859132107, 19.99746927611068870, 11.95042449705224819 ) ) ;
#2071=CARTESIAN_POINT ( 'NONE',  ( 22.92515349615029407, 19.68371071013345741, 13.00425721518307753 ) ) ;
#2079=CARTESIAN_POINT ( 'NONE',  ( 19.38642580597931087, 17.15576104669793267, 13.00425794126423362 ) ) ;
#2091=CARTESIAN_POINT ( 'NONE',  ( -1.449747468305836229, 33.50000000000000000, 14.98437500000000711 ) ) ;
#2094=CARTESIAN_POINT ( 'NONE',  ( 1.449747468305833120, 33.50000000000000000, 14.82812500000000178 ) ) ;
#2097=CARTESIAN_POINT ( 'NONE',  ( -1.035533905932742638, 32.50000000000000000, 16.23437500000000355 ) ) ;
#2105=MECHANICAL_DESIGN_GEOMETRIC_PRESENTATION_REPRESENTATION('',(#6704),#8842);
#2118=CARTESIAN_POINT ( 'NONE',  ( 22.83430298279833437, 18.47273307877622983, 10.95195840513859231 ) ) ;
#2124=CARTESIAN_POINT ( 'NONE',  ( 2.500000000000007550, 31.03553390593274486, 14.67187500000000178 ) ) ;
#2126=ORIENTED_EDGE ( 'NONE', *, *, #6854, .T. ) ;
#2128=CARTESIAN_POINT ( 'NONE',  ( 23.59820535295391508, 19.10314065948846718, 10.95195840513859231 ) ) ;
#2130=CARTESIAN_POINT ( 'NONE',  ( 19.58285320134683261, 17.29236643726018130, 13.00425622583864715 ) ) ;
#2135=CARTESIAN_POINT ( 'NONE',  ( 16.16243297953557700, 18.78731448874862053, 13.21853671947355302 ) ) ;
#2142=CARTESIAN_POINT ( 'NONE',  ( -3.500000000000003109, 29.99999999999999645, 15.21875000000000355 ) ) ;
#2148=CARTESIAN_POINT ( 'NONE',  ( -3.467250377026234176, 29.51776231023078623, 17.49702953738633937 ) ) ;
#2149=CARTESIAN_POINT ( 'NONE',  ( 0.06616922564517314920, 33.50000000000000000, 14.65405841526694353 ) ) ;
#2164=CARTESIAN_POINT ( 'NONE',  ( 17.31910053175343478, 17.63064693655086757, 11.10566822806672427 ) ) ;
#2171=CARTESIAN_POINT ( 'NONE',  ( -2.500000000000005773, 29.99999999999999645, 13.96875000000000355 ) ) ;
#2173=CARTESIAN_POINT ( 'NONE',  ( 22.95140240311772573, 18.55416269319264444, 10.95195840513845553 ) ) ;
#2176=CARTESIAN_POINT ( 'NONE',  ( 21.54797068462080745, 18.65933514708097007, 13.00425721518307576 ) ) ;
#2183=CARTESIAN_POINT ( 'NONE',  ( 18.83452698454826901, 16.95224361855724737, 13.01423506301239819 ) ) ;
#2188=CARTESIAN_POINT ( 'NONE',  ( -3.500000000000003553, 31.44974746830583356, 13.89062500000000355 ) ) ;
#2193=CARTESIAN_POINT ( 'NONE',  ( 1.720978244806812496, 28.18544433887406342, 16.68530841526694175 ) ) ;
#2214=CLOSED_SHELL ( 'NONE', ( #1051, #3862, #5210, #5185, #7508, #1194, #1689, #4401 ) ) ;
#2215=CARTESIAN_POINT ( 'NONE',  ( 17.36588923991300604, 17.58385822839129986, 12.10347664333366247 ) ) ;
#2223=CARTESIAN_POINT ( 'NONE',  ( -2.500000000000004441, 28.96446609406725159, 15.29687500000000178 ) ) ;
#2227=CARTESIAN_POINT ( 'NONE',  ( 19.12295744889739879, 19.47009535162641569, 11.95042449705107224 ) ) ;
#2229=AXIS2_PLACEMENT_3D ( 'NONE', #7271, #10770, #6543 ) ;
#2232=CARTESIAN_POINT ( 'NONE',  ( 18.83452698454826901, 16.95224361855724737, 13.01423506301239819 ) ) ;
#2240=CARTESIAN_POINT ( 'NONE',  ( 22.11805565807571128, 22.55986279155152374, 12.00579112326941988 ) ) ;
#2246=CARTESIAN_POINT ( 'NONE',  ( -3.500000000000001332, 29.93383077435482065, 14.22094158473306535 ) ) ;
#2252=CARTESIAN_POINT ( 'NONE',  ( -1.720978244806810498, 31.81455566112594013, 16.06030841526693820 ) ) ;
#2255=CARTESIAN_POINT ( 'NONE',  ( 16.74199038347050816, 18.20775708483493460, 12.16198771834506509 ) ) ;
#2256=CARTESIAN_POINT ( 'NONE',  ( -2.500000000000004441, 28.96446609406725514, 14.04687500000000355 ) ) ;
#2272=CARTESIAN_POINT ( 'NONE',  ( 21.07346791105437589, 22.52558620363005915, 11.00732503135576401 ) ) ;
#2286=CARTESIAN_POINT ( 'NONE',  ( 20.62599888145302529, 16.93661977612163128, 10.95195840513859231 ) ) ;
#2288=CARTESIAN_POINT ( 'NONE',  ( 22.99351140629659795, 23.33806509665494389, 12.94889058896590583 ) ) ;
#2295=CARTESIAN_POINT ( 'NONE',  ( 19.72936730704260810, 17.39430066254168139, 13.00425721518307576 ) ) ;
#2299=CARTESIAN_POINT ( 'NONE',  ( -0.06616922564517661864, 33.50000000000000000, 13.90844158473306713 ) ) ;
#2304=CARTESIAN_POINT ( 'NONE',  ( 1.814555661125939467, 31.72097824480680828, 15.74780841526694175 ) ) ;
#2314=CARTESIAN_POINT ( 'NONE',  ( -1.734723475976807094E-15, 33.50000000000000000, 13.65625000000000355 ) ) ;
#2318=CARTESIAN_POINT ( 'NONE',  ( 22.88317621546045189, 19.71992003298075957, 12.00579112326941988 ) ) ;
#2329=CARTESIAN_POINT ( 'NONE',  ( 18.76115673388714455, 17.03897527867736983, 11.01746215567925269 ) ) ;
#2334=CARTESIAN_POINT ( 'NONE',  ( 23.01143949934618504, 18.46103507366711227, 12.94889058896576906 ) ) ;
#2339=CARTESIAN_POINT ( 'NONE',  ( -3.500000000000003553, 31.44974746830583356, 13.89062500000000355 ) ) ;
#2341=CARTESIAN_POINT ( 'NONE',  ( 22.32737213215407479, 19.20149278331202325, 13.00425721518307576 ) ) ;
#2347=CARTESIAN_POINT ( 'NONE',  ( 3.527408190673962274, 28.61642175733934934, 13.51781658473306713 ) ) ;
#2348=DIRECTION ( 'NONE',  ( -0.7071067811865405783, -0.7071067811865545671, 0.000000000000000000 ) ) ;
#2354=CARTESIAN_POINT ( 'NONE',  ( 2.521662442312485819, 32.42808502599335441, 15.74780841526694175 ) ) ;
#2368=CARTESIAN_POINT ( 'NONE',  ( 20.28019557727208166, 19.74811736329550982, 11.00732503135576401 ) ) ;
#2380=CARTESIAN_POINT ( 'NONE',  ( 16.89796509758404852, 18.05178237072099989, 12.14735994959144350 ) ) ;
#2386=CARTESIAN_POINT ( 'NONE',  ( 21.33873319047917150, 17.29751440752404434, 12.94889058896590583 ) ) ;
#2391=ORIENTED_EDGE ( 'NONE', *, *, #10554, .F. ) ;
#2393=CARTESIAN_POINT ( 'NONE',  ( -3.500000000000005329, 30.06616922564516869, 14.96655841526694175 ) ) ;
#2397=CARTESIAN_POINT ( 'NONE',  ( 21.41520517525563605, 22.70178780811528441, 13.00425721518307753 ) ) ;
#2404=CARTESIAN_POINT ( 'NONE',  ( -1.515916693951010252, 33.47259180932604750, 15.23656658473306535 ) ) ;
#2406=EDGE_LOOP ( 'NONE', ( #1931, #8109, #8691, #3615 ) ) ;
#2415=CARTESIAN_POINT ( 'NONE',  ( 18.10462311893278553, 17.05669763433401087, 12.04589798090090902 ) ) ;
#2424=CARTESIAN_POINT ( 'NONE',  ( -1.449747468305830678, 26.49999999999999289, 14.20312500000000355 ) ) ;
#2425=CARTESIAN_POINT ( 'NONE',  ( -1.767766952966370209, 28.23223304703362402, 14.12500000000000355 ) ) ;
#2429=CARTESIAN_POINT ( 'NONE',  ( 21.42382487881899777, 22.58916947935290764, 11.00732503135576401 ) ) ;
#2444=CARTESIAN_POINT ( 'NONE',  ( 17.82405332881840110, 17.21173750719964346, 11.06307126761931769 ) ) ;
#2446=SURFACE_STYLE_FILL_AREA ( #4059 ) ;
#2449=CARTESIAN_POINT ( 'NONE',  ( 19.79543838746868190, 16.23930471839911149, 12.94973781945951785 ) ) ;
#2453=COLOUR_RGB ( '', 0.40784314, 0.44705882, 0.49803922) ;
#2457=PRODUCT_DEFINITION_CONTEXT ( 'detailed design', #4593, 'design' ) ;
#2460=CARTESIAN_POINT ( 'NONE',  ( 2.474873734152922111, 27.52512626584708144, 14.43750000000000178 ) ) ;
#2462=CARTESIAN_POINT ( 'NONE',  ( 22.73223279825284848, 19.49146071982302075, 13.00425721518307753 ) ) ;
#2463=CARTESIAN_POINT ( 'NONE',  ( 21.30711663910541276, 17.34296610691914253, 11.95042449705224819 ) ) ;
#2467=CARTESIAN_POINT ( 'NONE',  ( -2.428085025993349078, 27.47833755768751374, 13.12719158473306535 ) ) ;
#2475=CARTESIAN_POINT ( 'NONE',  ( 19.84380896203909828, 21.37294244821887546, 12.00579112326902731 ) ) ;
#2476=CARTESIAN_POINT ( 'NONE',  ( 2.500000000000007550, 31.03553390593274486, 14.67187500000000178 ) ) ;
#2484=CARTESIAN_POINT ( 'NONE',  ( 1.035533905932737975, 32.50000000000000711, 13.57812500000000178 ) ) ;
#2488=CARTESIAN_POINT ( 'NONE',  ( 20.00651627240589647, 19.97666299463432438, 12.00579112326824216 ) ) ;
#2498=CARTESIAN_POINT ( 'NONE',  ( 19.92593468680574986, 17.66592327340909918, 11.00732503135576401 ) ) ;
#2501=CARTESIAN_POINT ( 'NONE',  ( 21.07893270796819962, 17.11679519544646411, 12.94889058896590583 ) ) ;
#2509=CARTESIAN_POINT ( 'NONE',  ( 1.383578242660657098, 33.52740819067396671, 12.58031658473306713 ) ) ;
#2511=CARTESIAN_POINT ( 'NONE',  ( 15.22014049957087956, 18.31539340636219393, 13.24059312800850030 ) ) ;
#2516=CARTESIAN_POINT ( 'NONE',  ( -1.767766952966375094, 31.76776695296636888, 15.06250000000000355 ) ) ;
#2548=CARTESIAN_POINT ( 'NONE',  ( 16.63280437751621577, 18.31694309078998018, 13.17442390236345595 ) ) ;
#2553=CARTESIAN_POINT ( 'NONE',  ( 22.60530603367148927, 19.52972610220585636, 11.00732503135576401 ) ) ;
#2560=CARTESIAN_POINT ( 'NONE',  ( 20.49609864019753402, 16.84626017008312360, 10.95195840513859231 ) ) ;
#2568=CARTESIAN_POINT ( 'NONE',  ( -2.474873734152920335, 32.47487373415291501, 16.31250000000000355 ) ) ;
#2569=AXIS2_PLACEMENT_3D ( 'NONE', #7253, #3189, #3038 ) ;
#2571=CARTESIAN_POINT ( 'NONE',  ( 19.78966864679935611, 21.38900865752197689, 13.00425721518248956 ) ) ;
#2576=CARTESIAN_POINT ( 'NONE',  ( 21.41951502703731691, 22.64547864373410135, 12.00579112326941988 ) ) ;
#2579=CARTESIAN_POINT ( 'NONE',  ( 2.500000000000010214, 28.96446609406726225, 15.76562500000000178 ) ) ;
#2590=CARTESIAN_POINT ( 'NONE',  ( 22.63806431670481700, 19.48506897666907989, 12.00579112326951758 ) ) ;
#2593=CARTESIAN_POINT ( 'NONE',  ( 2.500000000000007550, 31.03553390593274486, 15.92187500000000178 ) ) ;
#2599=VERTEX_POINT ( 'NONE', #3423 ) ;
#2611=CARTESIAN_POINT ( 'NONE',  ( 16.58601566935801586, 18.36373179894819074, 12.17661548709639696 ) ) ;
#2617=CARTESIAN_POINT ( 'NONE',  ( 22.69616945897178084, 19.53356342368596898, 12.00579112326941988 ) ) ;
#2622=CARTESIAN_POINT ( 'NONE',  ( 21.79510105275299026, 17.74985623046760708, 10.95195840513859231 ) ) ;
#2634=CARTESIAN_POINT ( 'NONE',  ( -1.449747468305836229, 33.50000000000000000, 14.98437500000000711 ) ) ;
#2636=CARTESIAN_POINT ( 'NONE',  ( 22.43871220627207563, 23.52649944903870249, 11.95042449705224819 ) ) ;
#2640=CARTESIAN_POINT ( 'NONE',  ( 21.51635413324704160, 18.70478684647606826, 12.00579112326941988 ) ) ;
#2643=CARTESIAN_POINT ( 'NONE',  ( -2.385244779468109755E-15, 32.50000000000000711, 16.15625000000000355 ) ) ;
#2673=CARTESIAN_POINT ( 'NONE',  ( 19.84380896203909828, 21.37294244821887546, 12.00579112326902731 ) ) ;
#2677=CARTESIAN_POINT ( 'NONE',  ( 23.79237391907785693, 22.55645663433636017, 11.95042449705224819 ) ) ;
#2684=CARTESIAN_POINT ( 'NONE',  ( 3.500000000000005329, 30.00000000000000000, 15.84375000000000355 ) ) ;
#2686=CARTESIAN_POINT ( 'NONE',  ( 21.33748252609158058, 23.71725136694109892, 12.94889058896590583 ) ) ;
#2689=CARTESIAN_POINT ( 'NONE',  ( 20.52771519157129987, 16.80080847068802541, 11.95042449705224819 ) ) ;
#2690=CARTESIAN_POINT ( 'NONE',  ( 20.43380676890320657, 22.25420293214091316, 12.00579112326941988 ) ) ;
#2693=CARTESIAN_POINT ( 'NONE',  ( -1.101703131577916883, 32.47259180932605460, 15.23656658473306535 ) ) ;
#2698=CARTESIAN_POINT ( 'NONE',  ( 18.27511531525127353, 17.01097670698189290, 12.03680973694848966 ) ) ;
#2702=CARTESIAN_POINT ( 'NONE',  ( 22.88317621546045189, 19.71992003298075957, 12.00579112326941988 ) ) ;
#2703=CARTESIAN_POINT ( 'NONE',  ( -2.385244779468109755E-15, 32.50000000000000711, 14.90625000000000355 ) ) ;
#2712=CARTESIAN_POINT ( 'NONE',  ( -1.035533905932742638, 32.50000000000000000, 16.23437500000000355 ) ) ;
#2713=CARTESIAN_POINT ( 'NONE',  ( 4.553649124439118623E-15, 27.49999999999999289, 15.53125000000000355 ) ) ;
#2726=ORIENTED_EDGE ( 'NONE', *, *, #6807, .T. ) ;
#2729=CARTESIAN_POINT ( 'NONE',  ( 19.32754978430113368, 16.15626933694376888, 10.95875375162450638 ) ) ;
#2736=CARTESIAN_POINT ( 'NONE',  ( 1.515916693951011140, 26.52740819067395250, 14.61156658473306713 ) ) ;
#2739=CARTESIAN_POINT ( 'NONE',  ( 20.52771519157129987, 16.80080847068802541, 11.95042449705224819 ) ) ;
#2743=CARTESIAN_POINT ( 'NONE',  ( 17.65010306112908722, 17.31038946799904465, 12.07741653513508417 ) ) ;
#2766=CARTESIAN_POINT ( 'NONE',  ( -0.9693646802875689472, 32.52740819067395961, 14.73218341526694175 ) ) ;
#2768=CARTESIAN_POINT ( 'NONE',  ( -1.767766952966375094, 31.76776695296636888, 16.31250000000000355 ) ) ;
#2788=CARTESIAN_POINT ( 'NONE',  ( 15.98809489411982199, 17.54743901181251786, 11.16417930307855677 ) ) ;
#2796=CARTESIAN_POINT ( 'NONE',  ( 0.06616922564517943584, 27.49999999999998934, 14.53344158473306535 ) ) ;
#2798=CARTESIAN_POINT ( 'NONE',  ( 21.04731615659443733, 17.16224689484156585, 11.95042449705224819 ) ) ;
#2802=CARTESIAN_POINT ( 'NONE',  ( 16.89796509758404852, 18.05178237072099989, 12.14735994959144350 ) ) ;
#2821=CARTESIAN_POINT ( 'NONE',  ( 3.500000000000005329, 30.00000000000000000, 14.59375000000000178 ) ) ;
#2826=CARTESIAN_POINT ( 'NONE',  ( 1.035533905932737975, 32.50000000000000711, 14.82812500000000178 ) ) ;
#2844=( BOUNDED_CURVE ( )  B_SPLINE_CURVE ( 2, ( #6630, #8309, #2314, #3254, #10811, #10036, #1429, #10755, #4824, #2424, #7421, #640, #9978, #6527, #5812, #5705, #9927, #9038, #5754, #3196, #578, #6577, #3974, #9084, #9139, #1479, #1535, #8253, #4938, #213, #1787, #5176, #272, #7730, #6002, #3454, #1049, #7000, #3612, #2002, #883 ),
 .UNSPECIFIED., .F., .T. ) 
 B_SPLINE_CURVE_WITH_KNOTS ( ( 3, 2, 2, 2, 2, 2, 2, 2, 2, 2, 2, 2, 2, 2, 2, 2, 2, 2, 2, 2, 3 ),
 ( -1.684088607864716175E-18, 0.04166666666666666435, 0.08333333333333332871, 0.1250000000000000000, 0.1666666666666666574, 0.2083333333333333148, 0.2500000000000000000, 0.2916666666666666852, 0.3333333333333333148, 0.3750000000000000000, 0.4166666666666666297, 0.4583333333333333148, 0.5000000000000000000, 0.5416666666666666297, 0.5833333333333333703, 0.6250000000000000000, 0.6666666666666666297, 0.7083333333333334814, 0.7500000000000000000, 0.7916666666666666297, 0.8001047462599640836 ),
 .UNSPECIFIED. ) 
 CURVE ( )  GEOMETRIC_REPRESENTATION_ITEM ( )  RATIONAL_B_SPLINE_CURVE ( ( 1.000000000000000000, 0.9238795325112867385, 1.000000000000000000, 0.9238795325112867385, 1.000000000000000000, 0.9238795325112867385, 1.000000000000000000, 0.9238795325112867385, 1.000000000000000000, 0.9238795325112867385, 1.000000000000000000, 0.9238795325112867385, 1.000000000000000000, 0.9238795325112867385, 1.000000000000000000, 0.9238795325112867385, 1.000000000000000000, 0.9238795325112867385, 1.000000000000000000, 0.9238795325112867385, 1.000000000000000000, 0.9238795325112867385, 1.000000000000000000, 0.9238795325112867385, 1.000000000000000000, 0.9238795325112867385, 1.000000000000000000, 0.9238795325112867385, 1.000000000000000000, 0.9238795325112867385, 1.000000000000000000, 0.9238795325112867385, 1.000000000000000000, 0.9238795325112867385, 1.000000000000000000, 0.9238795325112867385, 1.000000000000000000, 0.9238795325112867385, 1.000000000000000000, 0.9845845464796294522, 0.9754127805002987817 ) ) 
 REPRESENTATION_ITEM ( '' )  );
#2846=CARTESIAN_POINT ( 'NONE',  ( 23.74733166794916528, 22.52239063326518220, 10.95195840513859231 ) ) ;
#2853=CARTESIAN_POINT ( 'NONE',  ( -2.500000000000003997, 29.93383077435482065, 14.22094158473306535 ) ) ;
#2855=CARTESIAN_POINT ( 'NONE',  ( 18.94130700685887447, 16.00034706198404066, 11.96718634320919250 ) ) ;
#2858=CARTESIAN_POINT ( 'NONE',  ( 21.04196501824306864, 22.63405165899350635, 13.00425721518307753 ) ) ;
#2870=CARTESIAN_POINT ( 'NONE',  ( -1.449747468305830678, 26.49999999999999289, 15.45312500000000178 ) ) ;
#2875=CARTESIAN_POINT ( 'NONE',  ( 2.527408190673967159, 30.96936468028756906, 15.66968341526694175 ) ) ;
#2876=CARTESIAN_POINT ( 'NONE',  ( 4.553649124439118623E-15, 27.49999999999999289, 14.28125000000000355 ) ) ;
#2877=CARTESIAN_POINT ( 'NONE',  ( 23.04535143233503192, 19.92821688535955360, 12.00579112326941988 ) ) ;
#2897=CARTESIAN_POINT ( 'NONE',  ( 17.40659673382103989, 17.54313596447427770, 11.09746175923963918 ) ) ;
#2904=CARTESIAN_POINT ( 'NONE',  ( 1.767766952966372429, 31.76776695296637598, 14.75000000000000355 ) ) ;
#2906=CARTESIAN_POINT ( 'NONE',  ( 19.86895450806392560, 16.41003605044161162, 10.95195963068177392 ) ) ;
#2910=CARTESIAN_POINT ( 'NONE',  ( 20.76856923708738734, 18.11717751085002703, 13.00425721518307576 ) ) ;
#2917=CARTESIAN_POINT ( 'NONE',  ( 16.94475380574361623, 18.00499366256143219, 13.14516836485838169 ) ) ;
#2926=CARTESIAN_POINT ( 'NONE',  ( 3.527408190673964494, 31.38357824266065776, 16.91968341526693820 ) ) ;
#2931=CARTESIAN_POINT ( 'NONE',  ( 1.814555661125939467, 31.72097824480680828, 14.49780841526694175 ) ) ;
#2932=CARTESIAN_POINT ( 'NONE',  ( 1.767766952966372429, 31.76776695296637598, 16.00000000000000355 ) ) ;
#2933=CARTESIAN_POINT ( 'NONE',  ( 19.69775075566884226, 17.43975236193677603, 12.00579112326941988 ) ) ;
#2951=CARTESIAN_POINT ( 'NONE',  ( 22.95140240311772573, 18.55416269319264444, 10.95195840513845553 ) ) ;
#2956=VERTEX_POINT ( 'NONE', #9912 ) ;
#2959=CARTESIAN_POINT ( 'NONE',  ( 2.527408190673965382, 29.03063531971243449, 13.51781658473306713 ) ) ;
#2963=CARTESIAN_POINT ( 'NONE',  ( 18.90462188152790901, 16.04371289204410189, 10.96879988954262153 ) ) ;
#2966=CARTESIAN_POINT ( 'NONE',  ( 19.38445574543743177, 22.63941596627307362, 11.95042449705263898 ) ) ;
#2968=CARTESIAN_POINT ( 'NONE',  ( 19.38642580597931087, 17.15576104669793267, 13.00425794126423362 ) ) ;
#2975=CARTESIAN_POINT ( 'NONE',  ( 21.54797068462080745, 18.65933514708097007, 13.00425721518307576 ) ) ;
#2976=B_SPLINE_CURVE_WITH_KNOTS ( 'NONE', 3,
 ( #7687, #3, #6786, #6015, #7570, #60, #3465, #8458, #7629, #10240, #9400, #1798, #5187, #8568, #950, #5023, #10295, #7744, #121, #3520, #6908, #2689, #8342, #10071, #2463, #5846, #9229, #1626, #775, #4182, #1233, #5349, #177, #7803, #1060, #5402, #7852, #3573, #1006, #5241, #7907, #4471, #6116, #7172, #10515, #1116, #2966, #2013, #226, #8786, #10568, #337 ),
 .UNSPECIFIED., .F., .F.,
 ( 4, 2, 2, 2, 2, 2, 2, 2, 2, 2, 2, 2, 2, 2, 2, 2, 2, 2, 2, 2, 2, 2, 2, 2, 2, 4 ),
 ( 0.05059550242215560267, 0.08415034466753366915, 0.1009277657902227232, 0.1177051869129117356, 0.1353321994545649831, 0.1529592119962182029, 0.1882132370795247256, 0.2234672621628312206, 0.2410942747044844681, 0.2587212872461377433, 0.2827395206008364026, 0.3067577539555350064, 0.3547942206649323249, 0.4028306873743295879, 0.4268489207290283027, 0.4508671540837269065, 0.4680275555186104164, 0.4851879569534939263, 0.5195087598232610571, 0.5881503655627953187, 0.6567919713023293582, 0.7254335770418635088, 0.7940751827813975483, 0.8627167885209316989, 0.9313583942604659605, 1.000000000000000000 ),
 .UNSPECIFIED. ) ;
#2984=CARTESIAN_POINT ( 'NONE',  ( 3.903127820947815962E-15, 26.49999999999999289, 15.53125000000000355 ) ) ;
#2987=CARTESIAN_POINT ( 'NONE',  ( -3.500000000000005329, 30.06616922564516869, 17.46655841526694175 ) ) ;
#2990=CARTESIAN_POINT ( 'NONE',  ( 2.527408190673967159, 30.96936468028756906, 16.91968341526693820 ) ) ;
#2991=CARTESIAN_POINT ( 'NONE',  ( 19.35452611835372849, 17.20101589911864437, 12.00579185514580338 ) ) ;
#3006=CARTESIAN_POINT ( 'NONE',  ( 24.04035011313704118, 22.03839429810881612, 10.95195840513898666 ) ) ;
#3011=EDGE_LOOP ( 'NONE', ( #3530, #13, #10343, #1374 ) ) ;
#3012=CARTESIAN_POINT ( 'NONE',  ( -1.035533905932742638, 32.50000000000000000, 13.73437500000000533 ) ) ;
#3015=CARTESIAN_POINT ( 'NONE',  ( 23.74733166794916528, 22.52239063326518220, 10.95195840513859231 ) ) ;
#3017=( LENGTH_UNIT ( ) NAMED_UNIT ( * ) SI_UNIT ( .MILLI., .METRE. ) );
#3019=CARTESIAN_POINT ( 'NONE',  ( 22.13583660366028738, 22.61346442202890472, 13.00425721518307753 ) ) ;
#3026=CARTESIAN_POINT ( 'NONE',  ( 19.35452611835372849, 17.20101589911864437, 12.00579185514580338 ) ) ;
#3031=CARTESIAN_POINT ( 'NONE',  ( -1.515916693951010252, 33.47259180932604750, 12.73656658473306358 ) ) ;
#3036=CARTESIAN_POINT ( 'NONE',  ( 2.428085025993357071, 27.47833755768751374, 15.43530841526694175 ) ) ;
#3038=DIRECTION ( 'NONE',  ( 0.7512361908166128588, 0.6577071706380231975, 0.05536662621716938876 ) ) ;
#3054=CARTESIAN_POINT ( 'NONE',  ( 17.60432978939287452, 17.35624782240900288, 11.07951759511215606 ) ) ;
#3062=CARTESIAN_POINT ( 'NONE',  ( 19.48730207459018970, 19.05393922246432226, 11.95042449705224996 ) ) ;
#3065=CARTESIAN_POINT ( 'NONE',  ( 19.95752144772427528, 19.94857296576799754, 13.00425721518131184 ) ) ;
#3073=CARTESIAN_POINT ( 'NONE',  ( 17.91214753276079819, 17.12229137291643610, 13.05912755560225236 ) ) ;
#3078=CARTESIAN_POINT ( 'NONE',  ( 0.9693646802875628410, 32.52740819067395961, 12.58031658473306713 ) ) ;
#3083=EDGE_CURVE ( 'NONE', #2599, #7325, #10373, .T. ) ;
#3085=CARTESIAN_POINT ( 'NONE',  ( -1.720978244806810498, 31.81455566112594013, 14.81030841526694175 ) ) ;
#3088=CARTESIAN_POINT ( 'NONE',  ( -2.500000000000005773, 29.99999999999999645, 13.96875000000000355 ) ) ;
#3102=CARTESIAN_POINT ( 'NONE',  ( 19.05040816462259556, 17.06282649731835122, 12.00984920396035172 ) ) ;
#3115=CARTESIAN_POINT ( 'NONE',  ( 19.17195227357822773, 19.49818538049391492, 10.95195840513741636 ) ) ;
#3117=CARTESIAN_POINT ( 'NONE',  ( 20.68923198420054987, 16.84571637733143490, 12.94889058896590583 ) ) ;
#3124=CARTESIAN_POINT ( 'NONE',  ( 22.45328846257175925, 22.40877220821986171, 12.00579112326941988 ) ) ;
#3129=CARTESIAN_POINT ( 'NONE',  ( -1.101703131577916883, 32.47259180932605460, 13.98656658473306713 ) ) ;
#3134=CARTESIAN_POINT ( 'NONE',  ( -3.472591809326048384, 31.51591669395100936, 14.88843341526694353 ) ) ;
#3153=CARTESIAN_POINT ( 'NONE',  ( 22.45328846257175925, 22.40877220821986171, 12.00579112326941988 ) ) ;
#3165=CARTESIAN_POINT ( 'NONE',  ( 23.11946528304491011, 21.60344811844516499, 11.00732503135595941 ) ) ;
#3169=CARTESIAN_POINT ( 'NONE',  ( 19.76265562249496099, 16.28401831655332543, 11.95127577209155234 ) ) ;
#3174=CARTESIAN_POINT ( 'NONE',  ( 1.449747468305833120, 33.50000000000000000, 13.57812500000000178 ) ) ;
#3176=CARTESIAN_POINT ( 'NONE',  ( 23.68215991433358525, 19.03072201379386641, 12.94889058896590583 ) ) ;
#3182=CARTESIAN_POINT ( 'NONE',  ( 0.9693646802875628410, 32.52740819067395961, 13.83031658473306535 ) ) ;
#3183=CYLINDRICAL_SURFACE ( 'NONE', #7746, 0.4999999999999883982 ) ;
#3187=CARTESIAN_POINT ( 'NONE',  ( 1.814555661125939467, 31.72097824480680828, 14.49780841526694175 ) ) ;
#3189=DIRECTION ( 'NONE',  ( 0.6587175828649983744, -0.7523902883640206651, 4.024558464266192459E-16 ) ) ;
#3196=CARTESIAN_POINT ( 'NONE',  ( -1.449747468305836229, 33.50000000000000000, 14.98437500000000533 ) ) ;
#3202=CARTESIAN_POINT ( 'NONE',  ( 23.17052989764754756, 21.62756661655841839, 12.00579112326981246 ) ) ;
#3216=CARTESIAN_POINT ( 'NONE',  ( 16.11564427137601285, 18.83410319690818824, 12.22072830420661660 ) ) ;
#3217=( NAMED_UNIT ( * ) PLANE_ANGLE_UNIT ( ) SI_UNIT ( $, .RADIAN. ) );
#3220=CARTESIAN_POINT ( 'NONE',  ( 17.43584335925693196, 16.24128823292743817, 13.04062965360331106 ) ) ;
#3227=CARTESIAN_POINT ( 'NONE',  ( 3.500000000000007994, 29.93383077435482420, 15.59155841526693997 ) ) ;
#3233=CARTESIAN_POINT ( 'NONE',  ( 23.37401553338360571, 20.56828919810574519, 13.00425721518307753 ) ) ;
#3238=CARTESIAN_POINT ( 'NONE',  ( 3.472591809326047052, 31.51591669395100936, 13.67406658473306535 ) ) ;
#3239=FACE_OUTER_BOUND ( 'NONE', #2406, .T. ) ;
#3254=CARTESIAN_POINT ( 'NONE',  ( -1.449747468305836229, 33.50000000000000000, 13.73437500000000888 ) ) ;
#3255=CARTESIAN_POINT ( 'NONE',  ( -2.500000000000005773, 29.99999999999999645, 13.96875000000000355 ) ) ;
#3259=CARTESIAN_POINT ( 'NONE',  ( 18.62184541094303114, 16.98042197548449295, 12.02177981800743112 ) ) ;
#3269=CARTESIAN_POINT ( 'NONE',  ( 22.10027471249113162, 22.50626116107413921, 11.00732503135576401 ) ) ;
#3270=( LENGTH_UNIT ( ) NAMED_UNIT ( * ) SI_UNIT ( .MILLI., .METRE. ) );
#3276=CARTESIAN_POINT ( 'NONE',  ( 24.08125446323534291, 19.61299372598402613, 12.94889058896590761 ) ) ;
#3285=CARTESIAN_POINT ( 'NONE',  ( 3.903127820947815962E-15, 26.49999999999999289, 14.28125000000000355 ) ) ;
#3289=CARTESIAN_POINT ( 'NONE',  ( 21.07893270796819962, 17.11679519544646411, 12.94889058896590583 ) ) ;
#3297=CARTESIAN_POINT ( 'NONE',  ( -3.527408190673960053, 31.38357824266065066, 15.39281658473306358 ) ) ;
#3306=CARTESIAN_POINT ( 'NONE',  ( 19.85760542366876535, 20.31250532737884384, 12.00579112326941988 ) ) ;
#3307=CARTESIAN_POINT ( 'NONE',  ( 1.035533905932737975, 32.50000000000000711, 13.57812500000000533 ) ) ;
#3331=CARTESIAN_POINT ( 'NONE',  ( 18.27511531525127353, 17.01097670698189290, 12.03680973694848966 ) ) ;
#3336=CARTESIAN_POINT ( 'NONE',  ( 21.85833415550051484, 17.65895283167741425, 12.94889058896590583 ) ) ;
#3340=( GEOMETRIC_REPRESENTATION_CONTEXT ( 3 ) GLOBAL_UNCERTAINTY_ASSIGNED_CONTEXT ( ( #3649 ) ) GLOBAL_UNIT_ASSIGNED_CONTEXT ( ( #3017, #5006, #10832 ) ) REPRESENTATION_CONTEXT ( 'NONE', 'WORKASPACE' ) );
#3346=CARTESIAN_POINT ( 'NONE',  ( -3.500000000000005329, 30.06616922564516869, 16.21655841526694175 ) ) ;
#3349=CARTESIAN_POINT ( 'NONE',  ( 17.82816014985957054, 16.05830732944317418, 13.01541525850460168 ) ) ;
#3354=CARTESIAN_POINT ( 'NONE',  ( -2.500000000000004441, 28.96446609406725159, 14.04687500000000355 ) ) ;
#3364=CARTESIAN_POINT ( 'NONE',  ( 22.45328846257175925, 22.40877220821986171, 12.00579112326941988 ) ) ;
#3365=CARTESIAN_POINT ( 'NONE',  ( -1.767766952966375094, 31.76776695296636888, 16.31250000000000355 ) ) ;
#3389=CARTESIAN_POINT ( 'NONE',  ( 21.48473758187327931, 18.75023854587115935, 11.00732503135576401 ) ) ;
#3392=CARTESIAN_POINT ( 'NONE',  ( 20.65761543282678758, 16.89116807672653664, 11.95042449705224819 ) ) ;
#3400=CARTESIAN_POINT ( 'NONE',  ( -2.474873734152920335, 32.47487373415291501, 15.06250000000000355 ) ) ;
#3402=CARTESIAN_POINT ( 'NONE',  ( 23.26157621925297647, 18.63507786824203549, 12.94889058896600353 ) ) ;
#3406=CARTESIAN_POINT ( 'NONE',  ( 19.55162244606592381, 17.33808635661342024, 12.00579012602852735 ) ) ;
#3409=CARTESIAN_POINT ( 'NONE',  ( 2.500000000000007550, 31.03553390593274486, 14.67187500000000178 ) ) ;
#3413=EDGE_LOOP ( 'NONE', ( #6855, #1806 ) ) ;
#3418=CARTESIAN_POINT ( 'NONE',  ( 20.73695268571362504, 18.16262921024512167, 12.00579112326941988 ) ) ;
#3423=CARTESIAN_POINT ( 'NONE',  ( 15.87890888817147150, 17.65662501776163040, 12.17661548709639341 ) ) ;
#3441=CARTESIAN_POINT ( 'NONE',  ( 15.87890888817147150, 17.65662501776163040, 12.17661548709639341 ) ) ;
#3447=CARTESIAN_POINT ( 'NONE',  ( 23.17052989764754756, 21.62756661655841839, 12.00579112326981246 ) ) ;
#3452=CARTESIAN_POINT ( 'NONE',  ( 22.60611905166032898, 18.24656216730335601, 11.95042449705224819 ) ) ;
#3454=CARTESIAN_POINT ( 'NONE',  ( -1.449747468305836229, 33.50000000000000000, 16.23437500000000355 ) ) ;
#3460=CARTESIAN_POINT ( 'NONE',  ( 2.474873734152918558, 32.47487373415292211, 16.00000000000000355 ) ) ;
#3463=CARTESIAN_POINT ( 'NONE',  ( 15.17335179141131185, 18.36218211452176519, 12.24278471274156388 ) ) ;
#3465=CARTESIAN_POINT ( 'NONE',  ( 16.72700999897183038, 16.80849948458634557, 12.09707671258119888 ) ) ;
#3466=CARTESIAN_POINT ( 'NONE',  ( 17.86810043078960319, 17.16701444005803268, 12.06109941161078325 ) ) ;
#3469=CARTESIAN_POINT ( 'NONE',  ( -2.385244779468109755E-15, 32.50000000000000711, 13.65625000000000355 ) ) ;
#3502=CARTESIAN_POINT ( 'NONE',  ( 18.79784185921769790, 16.99560944861731215, 12.01584860934582366 ) ) ;
#3507=CARTESIAN_POINT ( 'NONE',  ( 16.86040243112223180, 16.67515725582037689, 11.08237315523004973 ) ) ;
#3516=CARTESIAN_POINT ( 'NONE',  ( -1.449747468305836229, 33.50000000000000000, 16.23437500000000355 ) ) ;
#3518=CARTESIAN_POINT ( 'NONE',  ( 17.78598590678423719, 16.10215687441832699, 12.01726674494117653 ) ) ;
#3520=CARTESIAN_POINT ( 'NONE',  ( 20.15426471261298147, 16.54100339847095213, 11.95042283504686154 ) ) ;
#3523=CARTESIAN_POINT ( 'NONE',  ( 22.29575558078030895, 19.24694448270711788, 12.00579112326941988 ) ) ;
#3526=CARTESIAN_POINT ( 'NONE',  ( -2.500000000000005773, 29.99999999999999645, 15.21875000000000355 ) ) ;
#3530=ORIENTED_EDGE ( 'NONE', *, *, #7024, .T. ) ;
#3533=CARTESIAN_POINT ( 'NONE',  ( 17.65010306112908722, 17.31038946799904465, 12.07741653513508417 ) ) ;
#3536=CARTESIAN_POINT ( 'NONE',  ( 22.82387490247590733, 19.65457484615246386, 12.00579112326941988 ) ) ;
#3545=CARTESIAN_POINT ( 'NONE',  ( 0.06616922564517249694, 32.50000000000000711, 17.15405841526694175 ) ) ;
#3561=CARTESIAN_POINT ( 'NONE',  ( 16.67998965505631404, 16.85551971246726310, 11.09929001438087148 ) ) ;
#3569=CARTESIAN_POINT ( 'NONE',  ( -1.515916693951010252, 33.47259180932604750, 15.23656658473306535 ) ) ;
#3571=CARTESIAN_POINT ( 'NONE',  ( 22.47621881040483771, 18.15620256126511478, 11.95042449705224819 ) ) ;
#3573=CARTESIAN_POINT ( 'NONE',  ( 24.32342464814431438, 20.41340561598360992, 11.95042449705224996 ) ) ;
#3574=CARTESIAN_POINT ( 'NONE',  ( 23.04535143233503192, 19.92821688535955360, 12.00579112326941988 ) ) ;
#3594=CARTESIAN_POINT ( 'NONE',  ( -1.035533905932742638, 32.50000000000000000, 14.98437500000000711 ) ) ;
#3595=CARTESIAN_POINT ( 'NONE',  ( -2.385244779468109755E-15, 32.50000000000000711, 14.90625000000000355 ) ) ;
#3611=CARTESIAN_POINT ( 'NONE',  ( 16.45601903647678910, 17.07951486945825792, 11.12029599681952519 ) ) ;
#3612=CARTESIAN_POINT ( 'NONE',  ( -3.500000000000003109, 29.99999999999999645, 16.46875000000000355 ) ) ;
#3615=ORIENTED_EDGE ( 'NONE', *, *, #3083, .F. ) ;
#3616=DIRECTION ( 'NONE',  ( -0.7055570967602537991, 0.7055570967602550203, 0.06616922564517474514 ) ) ;
#3618=CARTESIAN_POINT ( 'NONE',  ( 1.101703131577918438, 27.52740819067395606, 14.61156658473306713 ) ) ;
#3620=CARTESIAN_POINT ( 'NONE',  ( 23.64018263364375017, 19.06693133664117212, 11.95042449705224819 ) ) ;
#3624=CARTESIAN_POINT ( 'NONE',  ( 19.85760542366876535, 20.31250532737884384, 12.00579112326941988 ) ) ;
#3642=CARTESIAN_POINT ( 'NONE',  ( -3.500000000000003109, 29.99999999999999645, 16.46875000000000355 ) ) ;
#3647=CARTESIAN_POINT ( 'NONE',  ( -2.527408190673963162, 29.03063531971243094, 15.04468341526694175 ) ) ;
#3648=FACE_OUTER_BOUND ( 'NONE', #3929, .T. ) ;
#3649=UNCERTAINTY_MEASURE_WITH_UNIT (LENGTH_MEASURE( 1.000000000000000082E-05 ), #3017, 'distance_accuracy_value', 'NONE');
#3651=CIRCLE ( 'NONE', #2229, 0.4999999999999981681 ) ;
#3668=CARTESIAN_POINT ( 'NONE',  ( 16.30404126228686579, 18.64570620602049189, 11.20086348037537327 ) ) ;
#3675=CARTESIAN_POINT ( 'NONE',  ( 2.500000000000006661, 30.06616922564517580, 13.59594158473306358 ) ) ;
#3677=CARTESIAN_POINT ( 'NONE',  ( 24.09141472773967507, 22.06251279622207306, 11.95042449705264076 ) ) ;
#3681=CARTESIAN_POINT ( 'NONE',  ( 15.22014049957087956, 18.31539340636219393, 13.24059312800850030 ) ) ;
#3697=CARTESIAN_POINT ( 'NONE',  ( -3.500000000000002220, 28.55025253169416288, 15.29687500000000178 ) ) ;
#3702=CARTESIAN_POINT ( 'NONE',  ( -1.814555661125937247, 28.27902175519318817, 15.12280841526694353 ) ) ;
#3704=CARTESIAN_POINT ( 'NONE',  ( -1.035533905932742638, 32.50000000000000000, 13.73437500000000533 ) ) ;
#3705=CARTESIAN_POINT ( 'NONE',  ( 22.98009469009668138, 21.94211999725310491, 12.00579112326941988 ) ) ;
#3722=CARTESIAN_POINT ( 'NONE',  ( 23.31046218964701211, 18.81639786330068276, 10.95195840513859231 ) ) ;
#3728=CARTESIAN_POINT ( 'NONE',  ( -1.767766952966370209, 28.23223304703362402, 14.12500000000000355 ) ) ;
#3730=CARTESIAN_POINT ( 'NONE',  ( 18.92159813099251053, 21.64660971755233732, 10.95195840513820151 ) ) ;
#3734=CARTESIAN_POINT ( 'NONE',  ( 17.07425424873056130, 16.47910233548095604, 13.06769463237219320 ) ) ;
#3750=CARTESIAN_POINT ( 'NONE',  ( -0.06616922564517661864, 33.50000000000000000, 12.65844158473306535 ) ) ;
#3755=CARTESIAN_POINT ( 'NONE',  ( -0.9693646802875689472, 32.52740819067395961, 15.98218341526694175 ) ) ;
#3757=CARTESIAN_POINT ( 'NONE',  ( 1.035533905932743970, 27.49999999999999289, 15.60937500000000711 ) ) ;
#3778=CARTESIAN_POINT ( 'NONE',  ( 18.81733698050991777, 21.09051435711097966, 10.95195840513859231 ) ) ;
#3785=CARTESIAN_POINT ( 'NONE',  ( -2.527408190673963162, 30.96936468028755840, 14.14281658473306713 ) ) ;
#3787=CARTESIAN_POINT ( 'NONE',  ( 21.27550008773165047, 17.38841780631423362, 10.95195840513859231 ) ) ;
#3790=CARTESIAN_POINT ( 'NONE',  ( 16.94475380574361623, 18.00499366256143219, 13.14516836485838169 ) ) ;
#3792=PRESENTATION_STYLE_ASSIGNMENT (( #4577 ) ) ;
#3795=EDGE_LOOP ( 'NONE', ( #10714, #4454, #10763, #2391 ) ) ;
#3796=CARTESIAN_POINT ( 'NONE',  ( 20.17304365239387565, 21.99495017005343200, 12.00579112326981068 ) ) ;
#3802=CARTESIAN_POINT ( 'NONE',  ( 3.472591809326051937, 28.48408330604899419, 16.76343341526694175 ) ) ;
#3807=CARTESIAN_POINT ( 'NONE',  ( -2.521662442312483599, 27.57191497400664204, 15.12280841526694353 ) ) ;
#3808=CARTESIAN_POINT ( 'NONE',  ( -1.814555661125937247, 28.27902175519318817, 15.12280841526694353 ) ) ;
#3830=CARTESIAN_POINT ( 'NONE',  ( 16.06885556321644160, 18.88089190506775594, 11.22291988893967840 ) ) ;
#3837=CARTESIAN_POINT ( 'NONE',  ( 4.553649124439118623E-15, 27.49999999999999289, 14.28125000000000355 ) ) ;
#3840=CARTESIAN_POINT ( 'NONE',  ( 19.52895938645546536, 19.09041019265748673, 10.95195840513859586 ) ) ;
#3843=CARTESIAN_POINT ( 'NONE',  ( 19.71976556488538534, 21.01616815698335827, 13.00425721518307753 ) ) ;
#3853=CARTESIAN_POINT ( 'NONE',  ( 23.04535143233503192, 19.92821688535955360, 12.00579112326941988 ) ) ;
#3859=CARTESIAN_POINT ( 'NONE',  ( 2.474873734152922111, 27.52512626584708144, 14.43750000000000178 ) ) ;
#3862=ADVANCED_FACE ( 'NONE', ( #3239 ), #3183, .T. ) ;
#3867=CARTESIAN_POINT ( 'NONE',  ( -1.720978244806810498, 31.81455566112594013, 17.31030841526694175 ) ) ;
#3884=CARTESIAN_POINT ( 'NONE',  ( 22.26413902940654665, 19.29239618210221607, 11.00732503135576401 ) ) ;
#3893=CARTESIAN_POINT ( 'NONE',  ( 16.67998965505631404, 16.85551971246726310, 11.09929001438087148 ) ) ;
#3898=CARTESIAN_POINT ( 'NONE',  ( 23.02513694122459498, 21.97618599832468433, 13.00425721518307753 ) ) ;
#3904=CARTESIAN_POINT ( 'NONE',  ( 17.69587633286529282, 17.26453111358909354, 13.07531547515800874 ) ) ;
#3909=EDGE_CURVE ( 'NONE', #2599, #10270, #481, .T. ) ;
#3912=CARTESIAN_POINT ( 'NONE',  ( 0.06616922564517879746, 26.50000000000000000, 13.28344158473306713 ) ) ;
#3916=CARTESIAN_POINT ( 'NONE',  ( 0.9693646802875698354, 27.47259180932603684, 15.35718341526694530 ) ) ;
#3927=CARTESIAN_POINT ( 'NONE',  ( 1.767766952966372429, 31.76776695296637598, 13.50000000000000355 ) ) ;
#3929=EDGE_LOOP ( 'NONE', ( #5381, #4219, #2726, #343 ) ) ;
#3933=CARTESIAN_POINT ( 'NONE',  ( 22.44007493706583745, 19.34731747087121434, 12.00579112326928133 ) ) ;
#3942=CARTESIAN_POINT ( 'NONE',  ( 19.46525898981753855, 16.20608772750926718, 10.95621100456342312 ) ) ;
#3946=CARTESIAN_POINT ( 'NONE',  ( 22.45649315185626094, 23.58010107951569623, 12.94889058896590583 ) ) ;
#3953=CARTESIAN_POINT ( 'NONE',  ( 22.82387490247590733, 19.65457484615246386, 12.00579112326941988 ) ) ;
#3957=CARTESIAN_POINT ( 'NONE',  ( -1.383578242660655100, 26.47259180932604039, 14.45531658473306535 ) ) ;
#3959=EDGE_CURVE ( 'NONE', #10270, #8937, #5142, .T. ) ;
#3964=CARTESIAN_POINT ( 'NONE',  ( -1.383578242660661983, 33.52740819067396671, 14.73218341526694175 ) ) ;
#3974=CARTESIAN_POINT ( 'NONE',  ( -3.500000000000003109, 29.99999999999999645, 15.21875000000000355 ) ) ;
#3981=CARTESIAN_POINT ( 'NONE',  ( 23.33980466280999977, 20.94445964013513617, 12.00579112326902909 ) ) ;
#3991=CARTESIAN_POINT ( 'NONE',  ( -1.035533905932742638, 32.50000000000000000, 16.23437500000000355 ) ) ;
#3995=CARTESIAN_POINT ( 'NONE',  ( 21.87443830563928415, 19.02131736398618855, 11.00732503135576401 ) ) ;
#3998=CARTESIAN_POINT ( 'NONE',  ( 18.94130700685887447, 16.00034706198404066, 11.96718634320919250 ) ) ;
#4006=CARTESIAN_POINT ( 'NONE',  ( 3.472591809326051937, 28.48408330604899419, 15.51343341526694353 ) ) ;
#4009=CARTESIAN_POINT ( 'NONE',  ( 21.05771646464872404, 22.57981893131178452, 12.00579112326941988 ) ) ;
#4015=CARTESIAN_POINT ( 'NONE',  ( -3.527408190673960053, 31.38357824266065066, 12.89281658473306535 ) ) ;
#4020=CARTESIAN_POINT ( 'NONE',  ( -0.9693646802875689472, 32.52740819067395961, 14.73218341526694175 ) ) ;
#4023=CARTESIAN_POINT ( 'NONE',  ( 17.45361707773674809, 17.49611573659335662, 12.09524845743996657 ) ) ;
#4043=CARTESIAN_POINT ( 'NONE',  ( 21.51635413324704160, 18.70478684647606826, 12.00579112326941988 ) ) ;
#4056=EDGE_LOOP ( 'NONE', ( #1230, #9407, #4490, #6501 ) ) ;
#4058=CARTESIAN_POINT ( 'NONE',  ( 17.54702143963720928, 17.40274154661815587, 11.08429399133878057 ) ) ;
#4059=FILL_AREA_STYLE ('',( #7440 ) ) ;
#4062=CARTESIAN_POINT ( 'NONE',  ( 17.82816014985957054, 16.05830732944317418, 13.01541525850460168 ) ) ;
#4065=CARTESIAN_POINT ( 'NONE',  ( 20.23853826540680600, 19.71164639310234534, 12.00579112326941988 ) ) ;
#4067=CARTESIAN_POINT ( 'NONE',  ( 1.515916693951008254, 33.47259180932604750, 14.57593341526694175 ) ) ;
#4070=CARTESIAN_POINT ( 'NONE',  ( 18.97799213218983994, 15.95698123192398477, 12.96557279687576525 ) ) ;
#4074=CARTESIAN_POINT ( 'NONE',  ( 3.500000000000003997, 30.06616922564517580, 13.59594158473306358 ) ) ;
#4083=CARTESIAN_POINT ( 'NONE',  ( 17.36588923991300604, 17.58385822839129986, 12.10347664333366247 ) ) ;
#4095=CARTESIAN_POINT ( 'NONE',  ( 21.25655365073496839, 18.52406763439849513, 12.00579112326941988 ) ) ;
#4105=CARTESIAN_POINT ( 'NONE',  ( -1.767766952966375094, 31.76776695296636888, 16.31250000000000355 ) ) ;
#4108=CARTESIAN_POINT ( 'NONE',  ( 17.36588923991300604, 17.58385822839129986, 12.10347664333366247 ) ) ;
#4111=CARTESIAN_POINT ( 'NONE',  ( 19.44564476272491049, 19.01746825227115067, 12.94889058896590761 ) ) ;
#4118=CARTESIAN_POINT ( 'NONE',  ( 1.515916693951008254, 33.47259180932604750, 17.07593341526694530 ) ) ;
#4120=CARTESIAN_POINT ( 'NONE',  ( 19.80390141066272491, 20.29503604781401904, 13.00425721518307753 ) ) ;
#4125=CARTESIAN_POINT ( 'NONE',  ( -2.472591809326046608, 28.89829686842208289, 14.29906658473306358 ) ) ;
#4126=ORIENTED_EDGE ( 'NONE', *, *, #8787, .T. ) ;
#4128=ORIENTED_EDGE ( 'NONE', *, *, #8914, .T. ) ;
#4135=CARTESIAN_POINT ( 'NONE',  ( 1.767766952966372429, 31.76776695296637598, 13.50000000000000355 ) ) ;
#4146=CARTESIAN_POINT ( 'NONE',  ( 22.63806431670481700, 19.48506897666907989, 12.00579112326951758 ) ) ;
#4158=CARTESIAN_POINT ( 'NONE',  ( 17.79249663040192431, 17.21067465782413919, 12.06642298039558980 ) ) ;
#4159=SHAPE_REPRESENTATION_RELATIONSHIP ( 'NONE' , 'NONE' ,  #716, #7322 ) ;
#4164=CARTESIAN_POINT ( 'NONE',  ( 20.29953126043439227, 16.57463755921569515, 12.94889058896590583 ) ) ;
#4175=CARTESIAN_POINT ( 'NONE',  ( 3.500000000000005329, 30.00000000000000000, 14.59375000000000178 ) ) ;
#4177=CIRCLE ( 'NONE', #9855, 0.5000000000000013323 ) ;
#4179=CARTESIAN_POINT ( 'NONE',  ( 19.71976556488538534, 21.01616815698335827, 13.00425721518307753 ) ) ;
#4182=CARTESIAN_POINT ( 'NONE',  ( 22.86591953417209666, 18.42728137938113875, 11.95042449705224819 ) ) ;
#4186=CARTESIAN_POINT ( 'NONE',  ( 1.767766952966372429, 31.76776695296637598, 13.50000000000000355 ) ) ;
#4187=DIRECTION ( 'NONE',  ( -0.7055570967602625698, 0.7055570967602455834, 0.06616922564518108729 ) ) ;
#4196=CARTESIAN_POINT ( 'NONE',  ( 19.77604874367146692, 21.01153129092389094, 12.00579112326941988 ) ) ;
#4201=FACE_OUTER_BOUND ( 'NONE', #7113, .T. ) ;
#4219=ORIENTED_EDGE ( 'NONE', *, *, #839, .T. ) ;
#4223=CARTESIAN_POINT ( 'NONE',  ( 20.05583492806123758, 17.75628287944761396, 11.00732503135576401 ) ) ;
#4229=CARTESIAN_POINT ( 'NONE',  ( 20.23629815768686768, 16.66554095800588797, 10.95195840513859231 ) ) ;
#4239=CARTESIAN_POINT ( 'NONE',  ( 1.515916693951011140, 26.52740819067395250, 13.36156658473306535 ) ) ;
#4242=CARTESIAN_POINT ( 'NONE',  ( 20.39832466968983837, 22.29813831026750393, 13.00425721518307753 ) ) ;
#4247=CARTESIAN_POINT ( 'NONE',  ( -1.767766952966375094, 31.76776695296636888, 13.81250000000000355 ) ) ;
#4257=CARTESIAN_POINT ( 'NONE',  ( 20.47715220320264962, 17.98190999816754498, 12.00579112326941988 ) ) ;
#4258=CARTESIAN_POINT ( 'NONE',  ( 1.767766952966372429, 31.76776695296637598, 16.00000000000000355 ) ) ;
#4280=CARTESIAN_POINT ( 'NONE',  ( 22.63806431670481700, 19.48506897666907989, 12.00579112326951758 ) ) ;
#4283=CARTESIAN_POINT ( 'NONE',  ( 21.82671760412675610, 17.70440453107251244, 11.95042449705224819 ) ) ;
#4293=CARTESIAN_POINT ( 'NONE',  ( 2.521662442312487151, 27.57191497400665270, 14.68969158473306535 ) ) ;
#4295=CARTESIAN_POINT ( 'NONE',  ( 23.58716357997163016, 18.92604383881832675, 12.94889058896590583 ) ) ;
#4296=DIRECTION ( 'NONE',  ( 0.000000000000000000, 0.000000000000000000, 1.000000000000000000 ) ) ;
#4298=CARTESIAN_POINT ( 'NONE',  ( 17.79249663040192431, 17.21067465782413919, 12.06642298039558980 ) ) ;
#4301=DIRECTION ( 'NONE',  ( -0.7055570967602625698, 0.7055570967602456944, 0.06616922564518108729 ) ) ;
#4335=CARTESIAN_POINT ( 'NONE',  ( 22.44007493706583745, 19.34731747087121434, 12.00579112326928133 ) ) ;
#4339=CARTESIAN_POINT ( 'NONE',  ( 20.77365933115271446, 23.55783661745384094, 11.95042449705224819 ) ) ;
#4349=CARTESIAN_POINT ( 'NONE',  ( 3.500000000000003997, 30.06616922564517580, 13.59594158473306358 ) ) ;
#4352=CARTESIAN_POINT ( 'NONE',  ( 23.83741617020655212, 22.59052263540754524, 12.94889058896590583 ) ) ;
#4355=CARTESIAN_POINT ( 'NONE',  ( 22.82387490247590733, 19.65457484615246386, 12.00579112326941988 ) ) ;
#4365=CARTESIAN_POINT ( 'NONE',  ( 18.62184541094303114, 16.98042197548449295, 12.02177981800743112 ) ) ;
#4380=CARTESIAN_POINT ( 'NONE',  ( 1.814555661125939467, 31.72097824480680828, 16.99780841526693820 ) ) ;
#4381=CARTESIAN_POINT ( 'NONE',  ( -2.500000000000004441, 28.96446609406725159, 15.29687500000000178 ) ) ;
#4389=CARTESIAN_POINT ( 'NONE',  ( 15.87890888817147150, 17.65662501776163040, 12.17661548709639696 ) ) ;
#4401=ADVANCED_FACE ( 'NONE', ( #7129 ), #9576, .T. ) ;
#4403=CARTESIAN_POINT ( 'NONE',  ( 17.34774915531493278, 16.33073436721105054, 11.04457336562047765 ) ) ;
#4414=CARTESIAN_POINT ( 'NONE',  ( 1.383578242660657098, 33.52740819067396671, 13.83031658473306535 ) ) ;
#4416=CARTESIAN_POINT ( 'NONE',  ( 19.07396262421655919, 19.44200532275891291, 12.94889058896472811 ) ) ;
#4422=CARTESIAN_POINT ( 'NONE',  ( 1.035533905932737975, 32.50000000000000711, 16.07812500000000355 ) ) ;
#4441=CARTESIAN_POINT ( 'NONE',  ( 1.035533905932743970, 27.49999999999999289, 15.60937500000000711 ) ) ;
#4442=CARTESIAN_POINT ( 'NONE',  ( -1.035533905932742638, 32.50000000000000000, 14.98437500000000711 ) ) ;
#4454=ORIENTED_EDGE ( 'NONE', *, *, #3909, .F. ) ;
#4457=CARTESIAN_POINT ( 'NONE',  ( 20.52771519157129987, 16.80080847068802541, 11.95042449705224819 ) ) ;
#4466=CARTESIAN_POINT ( 'NONE',  ( -1.515916693951010252, 33.47259180932604750, 12.73656658473306358 ) ) ;
#4468=CARTESIAN_POINT ( 'NONE',  ( 19.36223501247343393, 16.11237126175916501, 11.95718771041564210 ) ) ;
#4471=CARTESIAN_POINT ( 'NONE',  ( 22.96512898726170704, 23.28924158689358848, 11.95042449705224819 ) ) ;
#4472=CARTESIAN_POINT ( 'NONE',  ( 20.17304365239387565, 21.99495017005343200, 12.00579112326981068 ) ) ;
#4479=CARTESIAN_POINT ( 'NONE',  ( 16.11564427137601285, 18.83410319690818824, 12.22072830420661660 ) ) ;
#4487=CARTESIAN_POINT ( 'NONE',  ( -3.505208318772512488, 29.79067687212226545, 17.48140433884295319 ) ) ;
#4490=ORIENTED_EDGE ( 'NONE', *, *, #9950, .T. ) ;
#4492=CARTESIAN_POINT ( 'NONE',  ( -1.101703131577911776, 27.52740819067395250, 15.20093341526694353 ) ) ;
#4493=CARTESIAN_POINT ( 'NONE',  ( 1.767766952966372429, 31.76776695296637598, 13.50000000000000355 ) ) ;
#4507=CARTESIAN_POINT ( 'NONE',  ( 19.25788680476432546, 17.21053220311310739, 11.00783986014182148 ) ) ;
#4514=CARTESIAN_POINT ( 'NONE',  ( -1.101703131577916883, 32.47259180932605460, 15.23656658473306535 ) ) ;
#4516=CARTESIAN_POINT ( 'NONE',  ( 23.54706165660595829, 18.96431965174070555, 11.95042449705224819 ) ) ;
#4520=CARTESIAN_POINT ( 'NONE',  ( 22.03595509826854126, 19.06622527062933870, 12.00579112326941988 ) ) ;
#4538=CARTESIAN_POINT ( 'NONE',  ( -2.428085025993355295, 32.52166244231248271, 17.31030841526694175 ) ) ;
#4543=CARTESIAN_POINT ( 'NONE',  ( -2.500000000000004441, 28.96446609406725159, 15.29687500000000178 ) ) ;
#4546=CARTESIAN_POINT ( 'NONE',  ( 20.00651627240589647, 19.97666299463432438, 12.00579112326824216 ) ) ;
#4563=CARTESIAN_POINT ( 'NONE',  ( 17.74785087444460885, 17.25574343990722070, 11.06843699004799397 ) ) ;
#4569=CARTESIAN_POINT ( 'NONE',  ( -2.494791681227495950, 29.73705052183845154, 15.48578750830907147 ) ) ;
#4572=CARTESIAN_POINT ( 'NONE',  ( 24.04035011313704118, 22.03839429810881612, 10.95195840513898666 ) ) ;
#4575=CARTESIAN_POINT ( 'NONE',  ( 23.22159451225019566, 21.65168511467167889, 13.00425721518366728 ) ) ;
#4577=SURFACE_STYLE_USAGE ( .BOTH. , #1175 ) ;
#4593=APPLICATION_CONTEXT ( 'automotive_design' ) ;
#4595=CARTESIAN_POINT ( 'NONE',  ( -3.456897879362375470, 29.45240795142740353, 16.49922112211940117 ) ) ;
#4602=CARTESIAN_POINT ( 'NONE',  ( -2.472591809326051937, 31.10170313157791000, 16.13843341526694530 ) ) ;
#4603=CARTESIAN_POINT ( 'NONE',  ( -2.500000000000004441, 28.96446609406725159, 14.04687500000000355 ) ) ;
#4619=CARTESIAN_POINT ( 'NONE',  ( 18.92159813099251053, 21.64660971755233732, 10.95195840513820151 ) ) ;
#4624=( BOUNDED_SURFACE ( )  B_SPLINE_SURFACE ( 3, 3, ( 
 ( #951, #5301, #8569, #6117, #2802, #7688, #8628, #61, #7014, #896, #2743, #4298, #3466, #9568, #10241, #8519, #5958, #1118, #5188, #122, #1007, #3406, #9347, #1966, #5350, #10402, #9455, #8734, #2640, #8686, #4520, #3523, #7804, #5, #6909, #4355, #10296, #3574, #6787, #6847, #6959, #9511, #10347, #1061, #10182, #2576, #1744, #2690, #4472, #6016, #5139, #3624, #9401, #1799 ),
 ( #6065, #10673, #9619, #4631, #3790, #10516, #1344, #1172, #1291, #8015, #9841, #8850, #8061, #387, #4685, #7173, #2232, #1234, #443, #10569, #2968, #2130, #7121, #7229, #10626, #9010, #2910, #5404, #2176, #2014, #285, #6279, #4744, #7279, #502, #6341, #2071, #1401, #9677, #9735, #8119, #4575, #3898, #8951, #3019, #5517, #2858, #8899, #7908, #5459, #3843, #7075, #3065, #6394 ),
 ( #3681, #9785, #5624, #5571, #6440, #10464, #6228, #8789, #7961, #338, #3734, #6722, #3220, #4062, #4960, #4843, #760, #6552, #8217, #2449, #9999, #9104, #4164, #10719, #3117, #2501, #2386, #3336, #661, #5777, #546, #4795, #2334, #7444, #9161, #1500, #4901, #10115, #3276, #1557, #1612, #6599, #1450, #2288, #3946, #8331, #5888, #602, #8276, #9274, #10835, #6659, #710, #4111 ),
 ( #7498, #8171, #5010, #10885, #10060, #5836, #7331, #9219, #8385, #6495, #5676, #9897, #7558, #9055, #9949, #10943, #3998, #7388, #10779, #3169, #5727, #6833, #1836, #4457, #3392, #9388, #8556, #4283, #6102, #5944, #3452, #5124, #10334, #6894, #6001, #8673, #7618, #6358, #10389, #10281, #212, #939, #2677, #8445, #1667, #10226, #4339, #6052, #1786, #5175, #6998, #164, #9440, #9497 ),
 ( #10172, #824, #5229, #2788, #9332, #7729, #3611, #109, #3561, #3507, #8614, #994, #4403, #7790, #6163, #1897, #6944, #2729, #5284, #5066, #1048, #7839, #4229, #2560, #6773, #1726, #8502, #2622, #882, #7673, #48, #2118, #2951, #425, #3722, #9719, #1328, #271, #6265, #5447, #1159, #3006, #2846, #6326, #9660, #485, #10506, #5505, #2057, #4619, #3778, #8773, #8888, #1278 ),
 ( #7060, #3830, #3668, #1955, #7949, #6384, #8936, #2164, #2897, #7110, #3054, #4563, #8836, #9773, #6217, #5556, #10611, #4670, #7159, #4507, #10553, #9555, #327, #8049, #8720, #4728, #7215, #8105, #5336, #1102, #1222, #3884, #7267, #8004, #10662, #375, #7892, #10451, #9602, #2000, #5388, #4881, #5710, #6581, #6480, #2429, #2272, #5663, #9984, #6536, #9933, #4781, #5612, #2368 ),
 ( #10928, #1434, #5761, #8994, #9203, #9145, #1540, #2215, #6428, #9089, #8367, #696, #4830, #1596, #8261, #3259, #1385, #3102, #8159, #746, #644, #1483, #4945, #9881, #5821, #8205, #9042, #4095, #4043, #10760, #4994, #534, #3933, #4146, #7427, #7539, #2318, #10817, #7318, #9827, #3981, #3202, #8314, #3153, #7482, #10706, #10870, #6640, #10044, #585, #7375, #807, #2488, #92 ) ),
 .UNSPECIFIED., .T., .F., .F. ) 
 B_SPLINE_SURFACE_WITH_KNOTS ( ( 4, 3, 4 ),
 ( 4, 2, 2, 2, 2, 2, 2, 2, 2, 2, 2, 2, 2, 2, 2, 2, 2, 2, 2, 2, 2, 2, 2, 2, 2, 2, 4 ),
 ( 0.000000000000000000, 0.5000000000000000000, 1.000000000000000000 ),
 ( 0.000000000000000000, 0.05059550242166081097, 0.08415034466705637040, 0.1009277657897541536, 0.1177051869124519229, 0.1353321994541143436, 0.1529592119957767782, 0.1882132370791016474, 0.2234672621624265165, 0.2410942747040889511, 0.2587212872457513857, 0.2827395206004625905, 0.3067577539551737398, 0.3547942206645960939, 0.4028306873740183924, 0.4268489207287295972, 0.4508671540834407465, 0.4680275555183331937, 0.4851879569532256964, 0.5195087598230107018, 0.5881503655625806015, 0.6567919713021505013, 0.7254335770417204010, 0.7940751827812903008, 0.8627167885208602005, 0.9313583942604301003, 1.000000000000000000 ),
 .UNSPECIFIED. ) 
 GEOMETRIC_REPRESENTATION_ITEM ( )  RATIONAL_B_SPLINE_SURFACE ( (
 ( 1.000000000000000000, 1.000000000000000000, 1.000000000000000000, 1.000000000000000000, 1.000000000000000000, 1.000000000000000000, 1.000000000000000000, 1.000000000000000000, 1.000000000000000000, 1.000000000000000000, 1.000000000000000000, 1.000000000000000000, 1.000000000000000000, 1.000000000000000000, 1.000000000000000000, 1.000000000000000000, 1.000000000000000000, 1.000000000000000000, 1.000000000000000000, 1.000000000000000000, 1.000000000000000000, 1.000000000000000000, 1.000000000000000000, 1.000000000000000000, 1.000000000000000000, 1.000000000000000000, 1.000000000000000000, 1.000000000000000000, 1.000000000000000000, 1.000000000000000000, 1.000000000000000000, 1.000000000000000000, 1.000000000000000000, 1.000000000000000000, 1.000000000000000000, 1.000000000000000000, 1.000000000000000000, 1.000000000000000000, 1.000000000000000000, 1.000000000000000000, 1.000000000000000000, 1.000000000000000000, 1.000000000000000000, 1.000000000000000000, 1.000000000000000000, 1.000000000000000000, 1.000000000000000000, 1.000000000000000000, 1.000000000000000000, 1.000000000000000000, 1.000000000000000000, 1.000000000000000000, 1.000000000000000000, 1.000000000000000000),
 ( 0.3333333333333333703, 0.3333333333333333703, 0.3333333333333333703, 0.3333333333333333703, 0.3333333333333333703, 0.3333333333333333703, 0.3333333333333333703, 0.3333333333333333703, 0.3333333333333333703, 0.3333333333333333703, 0.3333333333333333703, 0.3333333333333333703, 0.3333333333333333703, 0.3333333333333333703, 0.3333333333333333703, 0.3333333333333333703, 0.3333333333333333703, 0.3333333333333333703, 0.3333333333333333703, 0.3333333333333333703, 0.3333333333333333703, 0.3333333333333333703, 0.3333333333333333703, 0.3333333333333333703, 0.3333333333333333703, 0.3333333333333333703, 0.3333333333333333703, 0.3333333333333333703, 0.3333333333333333703, 0.3333333333333333703, 0.3333333333333333703, 0.3333333333333333703, 0.3333333333333333703, 0.3333333333333333703, 0.3333333333333333703, 0.3333333333333333703, 0.3333333333333333703, 0.3333333333333333703, 0.3333333333333333703, 0.3333333333333333703, 0.3333333333333333703, 0.3333333333333333703, 0.3333333333333333703, 0.3333333333333333703, 0.3333333333333333703, 0.3333333333333333703, 0.3333333333333333703, 0.3333333333333333703, 0.3333333333333333703, 0.3333333333333333703, 0.3333333333333333703, 0.3333333333333333703, 0.3333333333333333703, 0.3333333333333333703),
 ( 0.3333333333333333703, 0.3333333333333333703, 0.3333333333333333703, 0.3333333333333333703, 0.3333333333333333703, 0.3333333333333333703, 0.3333333333333333703, 0.3333333333333333703, 0.3333333333333333703, 0.3333333333333333703, 0.3333333333333333703, 0.3333333333333333703, 0.3333333333333333703, 0.3333333333333333703, 0.3333333333333333703, 0.3333333333333333703, 0.3333333333333333703, 0.3333333333333333703, 0.3333333333333333703, 0.3333333333333333703, 0.3333333333333333703, 0.3333333333333333703, 0.3333333333333333703, 0.3333333333333333703, 0.3333333333333333703, 0.3333333333333333703, 0.3333333333333333703, 0.3333333333333333703, 0.3333333333333333703, 0.3333333333333333703, 0.3333333333333333703, 0.3333333333333333703, 0.3333333333333333703, 0.3333333333333333703, 0.3333333333333333703, 0.3333333333333333703, 0.3333333333333333703, 0.3333333333333333703, 0.3333333333333333703, 0.3333333333333333703, 0.3333333333333333703, 0.3333333333333333703, 0.3333333333333333703, 0.3333333333333333703, 0.3333333333333333703, 0.3333333333333333703, 0.3333333333333333703, 0.3333333333333333703, 0.3333333333333333703, 0.3333333333333333703, 0.3333333333333333703, 0.3333333333333333703, 0.3333333333333333703, 0.3333333333333333703),
 ( 1.000000000000000000, 1.000000000000000000, 1.000000000000000000, 1.000000000000000000, 1.000000000000000000, 1.000000000000000000, 1.000000000000000000, 1.000000000000000000, 1.000000000000000000, 1.000000000000000000, 1.000000000000000000, 1.000000000000000000, 1.000000000000000000, 1.000000000000000000, 1.000000000000000000, 1.000000000000000000, 1.000000000000000000, 1.000000000000000000, 1.000000000000000000, 1.000000000000000000, 1.000000000000000000, 1.000000000000000000, 1.000000000000000000, 1.000000000000000000, 1.000000000000000000, 1.000000000000000000, 1.000000000000000000, 1.000000000000000000, 1.000000000000000000, 1.000000000000000000, 1.000000000000000000, 1.000000000000000000, 1.000000000000000000, 1.000000000000000000, 1.000000000000000000, 1.000000000000000000, 1.000000000000000000, 1.000000000000000000, 1.000000000000000000, 1.000000000000000000, 1.000000000000000000, 1.000000000000000000, 1.000000000000000000, 1.000000000000000000, 1.000000000000000000, 1.000000000000000000, 1.000000000000000000, 1.000000000000000000, 1.000000000000000000, 1.000000000000000000, 1.000000000000000000, 1.000000000000000000, 1.000000000000000000, 1.000000000000000000),
 ( 0.3333333333333333703, 0.3333333333333333703, 0.3333333333333333703, 0.3333333333333333703, 0.3333333333333333703, 0.3333333333333333703, 0.3333333333333333703, 0.3333333333333333703, 0.3333333333333333703, 0.3333333333333333703, 0.3333333333333333703, 0.3333333333333333703, 0.3333333333333333703, 0.3333333333333333703, 0.3333333333333333703, 0.3333333333333333703, 0.3333333333333333703, 0.3333333333333333703, 0.3333333333333333703, 0.3333333333333333703, 0.3333333333333333703, 0.3333333333333333703, 0.3333333333333333703, 0.3333333333333333703, 0.3333333333333333703, 0.3333333333333333703, 0.3333333333333333703, 0.3333333333333333703, 0.3333333333333333703, 0.3333333333333333703, 0.3333333333333333703, 0.3333333333333333703, 0.3333333333333333703, 0.3333333333333333703, 0.3333333333333333703, 0.3333333333333333703, 0.3333333333333333703, 0.3333333333333333703, 0.3333333333333333703, 0.3333333333333333703, 0.3333333333333333703, 0.3333333333333333703, 0.3333333333333333703, 0.3333333333333333703, 0.3333333333333333703, 0.3333333333333333703, 0.3333333333333333703, 0.3333333333333333703, 0.3333333333333333703, 0.3333333333333333703, 0.3333333333333333703, 0.3333333333333333703, 0.3333333333333333703, 0.3333333333333333703),
 ( 0.3333333333333333703, 0.3333333333333333703, 0.3333333333333333703, 0.3333333333333333703, 0.3333333333333333703, 0.3333333333333333703, 0.3333333333333333703, 0.3333333333333333703, 0.3333333333333333703, 0.3333333333333333703, 0.3333333333333333703, 0.3333333333333333703, 0.3333333333333333703, 0.3333333333333333703, 0.3333333333333333703, 0.3333333333333333703, 0.3333333333333333703, 0.3333333333333333703, 0.3333333333333333703, 0.3333333333333333703, 0.3333333333333333703, 0.3333333333333333703, 0.3333333333333333703, 0.3333333333333333703, 0.3333333333333333703, 0.3333333333333333703, 0.3333333333333333703, 0.3333333333333333703, 0.3333333333333333703, 0.3333333333333333703, 0.3333333333333333703, 0.3333333333333333703, 0.3333333333333333703, 0.3333333333333333703, 0.3333333333333333703, 0.3333333333333333703, 0.3333333333333333703, 0.3333333333333333703, 0.3333333333333333703, 0.3333333333333333703, 0.3333333333333333703, 0.3333333333333333703, 0.3333333333333333703, 0.3333333333333333703, 0.3333333333333333703, 0.3333333333333333703, 0.3333333333333333703, 0.3333333333333333703, 0.3333333333333333703, 0.3333333333333333703, 0.3333333333333333703, 0.3333333333333333703, 0.3333333333333333703, 0.3333333333333333703),
 ( 1.000000000000000000, 1.000000000000000000, 1.000000000000000000, 1.000000000000000000, 1.000000000000000000, 1.000000000000000000, 1.000000000000000000, 1.000000000000000000, 1.000000000000000000, 1.000000000000000000, 1.000000000000000000, 1.000000000000000000, 1.000000000000000000, 1.000000000000000000, 1.000000000000000000, 1.000000000000000000, 1.000000000000000000, 1.000000000000000000, 1.000000000000000000, 1.000000000000000000, 1.000000000000000000, 1.000000000000000000, 1.000000000000000000, 1.000000000000000000, 1.000000000000000000, 1.000000000000000000, 1.000000000000000000, 1.000000000000000000, 1.000000000000000000, 1.000000000000000000, 1.000000000000000000, 1.000000000000000000, 1.000000000000000000, 1.000000000000000000, 1.000000000000000000, 1.000000000000000000, 1.000000000000000000, 1.000000000000000000, 1.000000000000000000, 1.000000000000000000, 1.000000000000000000, 1.000000000000000000, 1.000000000000000000, 1.000000000000000000, 1.000000000000000000, 1.000000000000000000, 1.000000000000000000, 1.000000000000000000, 1.000000000000000000, 1.000000000000000000, 1.000000000000000000, 1.000000000000000000, 1.000000000000000000, 1.000000000000000000) ) ) 
 REPRESENTATION_ITEM ( '' )  SURFACE ( )  );
#4625=ORIENTED_EDGE ( 'NONE', *, *, #6854, .F. ) ;
#4626=CARTESIAN_POINT ( 'NONE',  ( -0.06616922564517727090, 32.50000000000000711, 13.90844158473306713 ) ) ;
#4628=CARTESIAN_POINT ( 'NONE',  ( 15.83366986443827962, 19.11607760386789323, 11.24497629747462568 ) ) ;
#4631=CARTESIAN_POINT ( 'NONE',  ( 16.78877909162549642, 18.16096837667994279, 13.15979613361243494 ) ) ;
#4637=CARTESIAN_POINT ( 'NONE',  ( 23.33980466280999977, 20.94445964013513617, 12.00579112326902909 ) ) ;
#4644=CARTESIAN_POINT ( 'NONE',  ( -3.467250377026234176, 29.51776231023078623, 17.49702953738633937 ) ) ;
#4650=CARTESIAN_POINT ( 'NONE',  ( 3.527408190673964494, 31.38357824266065776, 15.66968341526694175 ) ) ;
#4651=CARTESIAN_POINT ( 'NONE',  ( -0.9693646802875689472, 32.52740819067395961, 17.23218341526694530 ) ) ;
#4670=CARTESIAN_POINT ( 'NONE',  ( 19.01572293645009637, 17.10672457250295508, 11.01141524516921422 ) ) ;
#4677=CARTESIAN_POINT ( 'NONE',  ( 1.720978244806805169, 31.81455566112594013, 12.50219158473306358 ) ) ;
#4681=CARTESIAN_POINT ( 'NONE',  ( 22.83430298279833437, 18.47273307877622983, 10.95195840513859231 ) ) ;
#4685=CARTESIAN_POINT ( 'NONE',  ( 18.31593954903570776, 16.96748919427588831, 13.03503021400358541 ) ) ;
#4691=CARTESIAN_POINT ( 'NONE',  ( 17.17871587691444546, 17.77103159139232957, 13.12322671172946897 ) ) ;
#4699=CARTESIAN_POINT ( 'NONE',  ( -1.449747468305836229, 33.50000000000000000, 16.23437500000000355 ) ) ;
#4704=CARTESIAN_POINT ( 'NONE',  ( 2.472591809326055046, 28.89829686842209355, 16.76343341526694175 ) ) ;
#4728=CARTESIAN_POINT ( 'NONE',  ( 20.44553565182888732, 18.02736169756263962, 11.00732503135576401 ) ) ;
#4735=CARTESIAN_POINT ( 'NONE',  ( -2.500000000000005773, 29.99999999999999645, 15.21875000000000355 ) ) ;
#4739=CARTESIAN_POINT ( 'NONE',  ( 15.98809489411982199, 17.54743901181251786, 11.16417930307855677 ) ) ;
#4744=CARTESIAN_POINT ( 'NONE',  ( 22.47009348518006888, 19.30075366110858326, 13.00425721518280042 ) ) ;
#4751=CARTESIAN_POINT ( 'NONE',  ( 17.50063742165245984, 17.44909550871243198, 13.09303515564029397 ) ) ;
#4758=CARTESIAN_POINT ( 'NONE',  ( -3.527408190673960053, 31.38357824266065066, 14.14281658473306713 ) ) ;
#4764=CARTESIAN_POINT ( 'NONE',  ( -2.428085025993355295, 32.52166244231248271, 16.06030841526693820 ) ) ;
#4781=CARTESIAN_POINT ( 'NONE',  ( 19.91130943667480224, 20.32997460694367575, 11.00732503135576401 ) ) ;
#4785=DIRECTION ( 'NONE',  ( 0.7512361908166128588, 0.6577071706380231975, 0.05536662621716938876 ) ) ;
#4790=CARTESIAN_POINT ( 'NONE',  ( 16.61199375056689931, 16.92354015536430722, 11.10566822806672427 ) ) ;
#4795=CARTESIAN_POINT ( 'NONE',  ( 22.89753608554585540, 18.38182967998604056, 12.94889058896590583 ) ) ;
#4801=CARTESIAN_POINT ( 'NONE',  ( 19.32345233471135515, 17.12110500680467240, 13.00476395487764947 ) ) ;
#4807=CARTESIAN_POINT ( 'NONE',  ( -2.527408190673963162, 30.96936468028755840, 12.89281658473306535 ) ) ;
#4812=CARTESIAN_POINT ( 'NONE',  ( -1.814555661125937247, 28.27902175519318817, 16.37280841526694175 ) ) ;
#4814=CARTESIAN_POINT ( 'NONE',  ( 17.13192716875488131, 17.81782029955189728, 12.12541829646253078 ) ) ;
#4824=CARTESIAN_POINT ( 'NONE',  ( -2.474873734152916338, 27.52512626584707789, 14.12500000000000355 ) ) ;
#4830=CARTESIAN_POINT ( 'NONE',  ( 17.86810043078960319, 17.16701444005803268, 12.06109941161078325 ) ) ;
#4839=CARTESIAN_POINT ( 'NONE',  ( 20.70533613433985920, 18.20808090964021986, 11.00732503135576401 ) ) ;
#4843=CARTESIAN_POINT ( 'NONE',  ( 18.68606934758710025, 15.93178998805769453, 12.97541080761745924 ) ) ;
#4848=CARTESIAN_POINT ( 'NONE',  ( -2.428085025993355295, 32.52166244231248271, 16.06030841526693820 ) ) ;
#4851=CARTESIAN_POINT ( 'NONE',  ( 19.98916778955327800, 17.57501987461890991, 13.00425721518307576 ) ) ;
#4856=CARTESIAN_POINT ( 'NONE',  ( 2.472591809326049272, 31.10170313157791711, 13.67406658473306535 ) ) ;
#4862=CARTESIAN_POINT ( 'NONE',  ( 1.101703131577913553, 32.47259180932605460, 17.07593341526694530 ) ) ;
#4881=CARTESIAN_POINT ( 'NONE',  ( 23.11946528304491011, 21.60344811844516499, 11.00732503135595941 ) ) ;
#4896=CARTESIAN_POINT ( 'NONE',  ( 19.52039169078502212, 17.38380627596665562, 11.00732402621840578 ) ) ;
#4897=SURFACE_STYLE_USAGE ( .BOTH. , #10058 ) ;
#4901=CARTESIAN_POINT ( 'NONE',  ( 23.68215991433358525, 19.03072201379386641, 12.94889058896590583 ) ) ;
#4910=CARTESIAN_POINT ( 'NONE',  ( 3.527408190673964494, 31.38357824266065776, 16.91968341526693820 ) ) ;
#4912=CARTESIAN_POINT ( 'NONE',  ( 22.86397682584157565, 19.61629903322988966, 13.00425721518307753 ) ) ;
#4916=CARTESIAN_POINT ( 'NONE',  ( -1.515916693951010252, 33.47259180932604750, 13.98656658473306713 ) ) ;
#4925=( BOUNDED_SURFACE ( )  B_SPLINE_SURFACE ( 3, 2, ( 
 ( #4493, #6308, #5321, #3704, #6198, #7093, #197, #4603, #5266, #10484, #2876, #6248, #1985, #5371, #5428, #148, #1032, #9642, #3595, #4442, #6929, #10318, #1198, #4381, #8705, #7985, #2713, #3757, #6982, #7876, #10537, #9701, #2932, #7768, #10369, #2097, #2768, #6144, #250, #7043, #10431 ),
 ( #3187, #6514, #10647, #4020, #3085, #9074, #8034, #8918, #3808, #9918, #464, #3916, #10692, #9029, #7300, #6458, #2304, #9863, #5695, #9807, #2252, #5647, #8191, #1420, #4812, #5744, #1470, #1308, #2193, #4704, #7250, #2990, #9757, #4862, #10741, #4651, #3867, #8974, #6568, #5588, #567 ),
 ( #8088, #8239, #2149, #3964, #7352, #3134, #627, #7408, #10801, #407, #6369, #9968, #3036, #5538, #7198, #10594, #2354, #1258, #6411, #1365, #4764, #8142, #518, #8915, #7927, #300, #402, #10532, #6243, #3802, #10643, #2926, #5583, #9637, #5532, #1304, #4538, #1077, #1979, #4487, #4644 ),
 ( #8869, #7088, #7036, #5366, #1252, #2188, #5481, #10588, #10479, #8029, #6193, #6299, #3859, #9751, #2821, #2028, #7871, #10423, #5422, #2091, #9695, #7136, #2142, #3697, #7192, #2870, #2984, #8810, #1190, #6363, #6405, #9580, #8749, #244, #1131, #4699, #8081, #458, #3642, #7244, #4595 ),
 ( #9802, #7979, #3750, #3031, #351, #4015, #677, #1360, #2467, #6678, #3912, #8968, #9857, #2347, #4074, #3238, #10076, #8345, #2299, #4916, #5790, #4758, #2246, #619, #10015, #3957, #7402, #7458, #8136, #513, #7292, #5739, #10686, #5690, #10795, #2404, #7345, #3297, #9119, #9068, #1414 ),
 ( #1515, #3078, #9177, #5640, #9913, #4807, #10735, #6452, #9024, #6611, #10847, #8185, #561, #1465, #10901, #4856, #8290, #3182, #1573, #3129, #4972, #6508, #725, #4125, #7513, #6563, #9963, #8230, #1630, #7573, #9403, #1683, #10963, #5027, #8399, #2693, #5850, #7, #63, #779, #5190 ),
 ( #4186, #845, #3469, #10349, #4247, #6018, #5083, #3354, #7632, #8572, #6735, #9232, #8521, #7806, #124, #3409, #8631, #7691, #6067, #10129, #2516, #5905, #3526, #8461, #898, #9288, #6789, #1850, #10184, #2579, #5245, #6850, #5961, #4422, #2643, #9349, #1746, #10298, #10243, #1009, #1801 ) ),
 .UNSPECIFIED., .T., .F., .F. ) 
 B_SPLINE_SURFACE_WITH_KNOTS ( ( 4, 3, 4 ),
 ( 3, 2, 2, 2, 2, 2, 2, 2, 2, 2, 2, 2, 2, 2, 2, 2, 2, 2, 2, 2, 3 ),
 ( 0.000000000000000000, 0.5000000000000000000, 1.000000000000000000 ),
 ( 0.000000000000000000, 0.04166666666666666435, 0.08333333333333332871, 0.1250000000000000000, 0.1666666666666666574, 0.2083333333333333426, 0.2500000000000000000, 0.2916666666666666852, 0.3333333333333333148, 0.3750000000000000000, 0.4166666666666666852, 0.4583333333333333148, 0.5000000000000000000, 0.5416666666666666297, 0.5833333333333333703, 0.6250000000000000000, 0.6666666666666666297, 0.7083333333333333703, 0.7500000000000000000, 0.7916666666666666297, 0.8001047462599640836 ),
 .UNSPECIFIED. ) 
 GEOMETRIC_REPRESENTATION_ITEM ( )  RATIONAL_B_SPLINE_SURFACE ( (
 ( 1.000000000000000000, 0.9238795325112867385, 1.000000000000000000, 0.9238795325112867385, 1.000000000000000000, 0.9238795325112867385, 1.000000000000000000, 0.9238795325112867385, 1.000000000000000000, 0.9238795325112867385, 1.000000000000000000, 0.9238795325112867385, 1.000000000000000000, 0.9238795325112867385, 1.000000000000000000, 0.9238795325112867385, 1.000000000000000000, 0.9238795325112867385, 1.000000000000000000, 0.9238795325112867385, 1.000000000000000000, 0.9238795325112867385, 1.000000000000000000, 0.9238795325112867385, 1.000000000000000000, 0.9238795325112867385, 1.000000000000000000, 0.9238795325112867385, 1.000000000000000000, 0.9238795325112867385, 1.000000000000000000, 0.9238795325112867385, 1.000000000000000000, 0.9238795325112867385, 1.000000000000000000, 0.9238795325112867385, 1.000000000000000000, 0.9238795325112867385, 1.000000000000000000, 0.9845845464796294522, 0.9754127805002987817),
 ( 0.3333333333333333703, 0.3079598441704289313, 0.3333333333333333703, 0.3079598441704289313, 0.3333333333333333703, 0.3079598441704289313, 0.3333333333333333703, 0.3079598441704289313, 0.3333333333333333703, 0.3079598441704289313, 0.3333333333333333703, 0.3079598441704289313, 0.3333333333333333703, 0.3079598441704289313, 0.3333333333333333703, 0.3079598441704289313, 0.3333333333333333703, 0.3079598441704289313, 0.3333333333333333703, 0.3079598441704289313, 0.3333333333333333703, 0.3079598441704289313, 0.3333333333333333703, 0.3079598441704289313, 0.3333333333333333703, 0.3079598441704289313, 0.3333333333333333703, 0.3079598441704289313, 0.3333333333333333703, 0.3079598441704289313, 0.3333333333333333703, 0.3079598441704289313, 0.3333333333333333703, 0.3079598441704289313, 0.3333333333333333703, 0.3079598441704289313, 0.3333333333333333703, 0.3079598441704289313, 0.3333333333333333703, 0.3281948488265432062, 0.3251375935000996309),
 ( 0.3333333333333333703, 0.3079598441704289313, 0.3333333333333333703, 0.3079598441704289313, 0.3333333333333333703, 0.3079598441704289313, 0.3333333333333333703, 0.3079598441704289313, 0.3333333333333333703, 0.3079598441704289313, 0.3333333333333333703, 0.3079598441704289313, 0.3333333333333333703, 0.3079598441704289313, 0.3333333333333333703, 0.3079598441704289313, 0.3333333333333333703, 0.3079598441704289313, 0.3333333333333333703, 0.3079598441704289313, 0.3333333333333333703, 0.3079598441704289313, 0.3333333333333333703, 0.3079598441704289313, 0.3333333333333333703, 0.3079598441704289313, 0.3333333333333333703, 0.3079598441704289313, 0.3333333333333333703, 0.3079598441704289313, 0.3333333333333333703, 0.3079598441704289313, 0.3333333333333333703, 0.3079598441704289313, 0.3333333333333333703, 0.3079598441704289313, 0.3333333333333333703, 0.3079598441704289313, 0.3333333333333333703, 0.3281948488265432062, 0.3251375935000996309),
 ( 1.000000000000000000, 0.9238795325112867385, 1.000000000000000000, 0.9238795325112867385, 1.000000000000000000, 0.9238795325112867385, 1.000000000000000000, 0.9238795325112867385, 1.000000000000000000, 0.9238795325112867385, 1.000000000000000000, 0.9238795325112867385, 1.000000000000000000, 0.9238795325112867385, 1.000000000000000000, 0.9238795325112867385, 1.000000000000000000, 0.9238795325112867385, 1.000000000000000000, 0.9238795325112867385, 1.000000000000000000, 0.9238795325112867385, 1.000000000000000000, 0.9238795325112867385, 1.000000000000000000, 0.9238795325112867385, 1.000000000000000000, 0.9238795325112867385, 1.000000000000000000, 0.9238795325112867385, 1.000000000000000000, 0.9238795325112867385, 1.000000000000000000, 0.9238795325112867385, 1.000000000000000000, 0.9238795325112867385, 1.000000000000000000, 0.9238795325112867385, 1.000000000000000000, 0.9845845464796294522, 0.9754127805002987817),
 ( 0.3333333333333333703, 0.3079598441704289313, 0.3333333333333333703, 0.3079598441704289313, 0.3333333333333333703, 0.3079598441704289313, 0.3333333333333333703, 0.3079598441704289313, 0.3333333333333333703, 0.3079598441704289313, 0.3333333333333333703, 0.3079598441704289313, 0.3333333333333333703, 0.3079598441704289313, 0.3333333333333333703, 0.3079598441704289313, 0.3333333333333333703, 0.3079598441704289313, 0.3333333333333333703, 0.3079598441704289313, 0.3333333333333333703, 0.3079598441704289313, 0.3333333333333333703, 0.3079598441704289313, 0.3333333333333333703, 0.3079598441704289313, 0.3333333333333333703, 0.3079598441704289313, 0.3333333333333333703, 0.3079598441704289313, 0.3333333333333333703, 0.3079598441704289313, 0.3333333333333333703, 0.3079598441704289313, 0.3333333333333333703, 0.3079598441704289313, 0.3333333333333333703, 0.3079598441704289313, 0.3333333333333333703, 0.3281948488265432062, 0.3251375935000996309),
 ( 0.3333333333333333703, 0.3079598441704289313, 0.3333333333333333703, 0.3079598441704289313, 0.3333333333333333703, 0.3079598441704289313, 0.3333333333333333703, 0.3079598441704289313, 0.3333333333333333703, 0.3079598441704289313, 0.3333333333333333703, 0.3079598441704289313, 0.3333333333333333703, 0.3079598441704289313, 0.3333333333333333703, 0.3079598441704289313, 0.3333333333333333703, 0.3079598441704289313, 0.3333333333333333703, 0.3079598441704289313, 0.3333333333333333703, 0.3079598441704289313, 0.3333333333333333703, 0.3079598441704289313, 0.3333333333333333703, 0.3079598441704289313, 0.3333333333333333703, 0.3079598441704289313, 0.3333333333333333703, 0.3079598441704289313, 0.3333333333333333703, 0.3079598441704289313, 0.3333333333333333703, 0.3079598441704289313, 0.3333333333333333703, 0.3079598441704289313, 0.3333333333333333703, 0.3079598441704289313, 0.3333333333333333703, 0.3281948488265432062, 0.3251375935000996309),
 ( 1.000000000000000000, 0.9238795325112867385, 1.000000000000000000, 0.9238795325112867385, 1.000000000000000000, 0.9238795325112867385, 1.000000000000000000, 0.9238795325112867385, 1.000000000000000000, 0.9238795325112867385, 1.000000000000000000, 0.9238795325112867385, 1.000000000000000000, 0.9238795325112867385, 1.000000000000000000, 0.9238795325112867385, 1.000000000000000000, 0.9238795325112867385, 1.000000000000000000, 0.9238795325112867385, 1.000000000000000000, 0.9238795325112867385, 1.000000000000000000, 0.9238795325112867385, 1.000000000000000000, 0.9238795325112867385, 1.000000000000000000, 0.9238795325112867385, 1.000000000000000000, 0.9238795325112867385, 1.000000000000000000, 0.9238795325112867385, 1.000000000000000000, 0.9238795325112867385, 1.000000000000000000, 0.9238795325112867385, 1.000000000000000000, 0.9238795325112867385, 1.000000000000000000, 0.9845845464796294522, 0.9754127805002987817) ) ) 
 REPRESENTATION_ITEM ( '' )  SURFACE ( )  );
#4938=CARTESIAN_POINT ( 'NONE',  ( 2.474873734152922111, 27.52512626584708144, 15.68750000000000355 ) ) ;
#4945=CARTESIAN_POINT ( 'NONE',  ( 19.69775075566884226, 17.43975236193677603, 12.00579112326941988 ) ) ;
#4951=CARTESIAN_POINT ( 'NONE',  ( 19.86292016999849608, 19.38279280778333202, 11.97810781016083403 ) ) ;
#4957=CARTESIAN_POINT ( 'NONE',  ( 17.13192716875488131, 17.81782029955189728, 12.12541829646253078 ) ) ;
#4960=CARTESIAN_POINT ( 'NONE',  ( 18.11095311068464397, 15.98247068297658835, 13.00034071860445550 ) ) ;
#4966=CARTESIAN_POINT ( 'NONE',  ( -2.428085025993355295, 32.52166244231248271, 17.31030841526694175 ) ) ;
#4968=CARTESIAN_POINT ( 'NONE',  ( 18.68606934758710025, 15.93178998805769453, 12.97541080761745924 ) ) ;
#4972=CARTESIAN_POINT ( 'NONE',  ( -1.814555661125939912, 31.72097824480680117, 14.06469158473306358 ) ) ;
#4980=CARTESIAN_POINT ( 'NONE',  ( 19.35452611835372849, 17.20101589911864437, 12.00579185514580338 ) ) ;
#4989=( BOUNDED_SURFACE ( )  B_SPLINE_SURFACE ( 3, 2, ( 
 ( #6867, #2484, #10261, #5868, #692, #7476, #3255, #1591, #2425, #5042, #9199, #8362, #742, #1082, #5212, #9584, #8755, #2826, #1136, #3594, #9640, #8648, #1030, #4543, #249, #6981, #10317, #4441, #5320, #1934, #10368, #6247, #2034, #5265, #6307, #2712, #1818, #5370, #8704, #10536, #1984 ),
 ( #2931, #6197, #7764, #2766, #10427, #7931, #306, #3647, #3702, #4492, #7875, #10483, #7822, #7042, #7092, #2875, #5427, #8815, #1195, #3755, #8590, #4602, #9476, #6143, #196, #974, #9533, #7984, #7140, #354, #1871, #6087, #4380, #145, #3545, #6928, #669, #5783, #5682, #10067, #10593 ),
 ( #717, #4067, #7451, #10893, #5487, #406, #2393, #9060, #3807, #7197, #1506, #10840, #1455, #4006, #3227, #4650, #9169, #9756, #7505, #1257, #4848, #6604, #3346, #8222, #10005, #610, #1565, #7394, #8033, #8874, #9700, #4910, #769, #4118, #10786, #1620, #4966, #6668, #2987, #6367, #2148 ),
 ( #8282, #3174, #6557, #5843, #9954, #2339, #9226, #8337, #5731, #8393, #3285, #9109, #2460, #5018, #4175, #7564, #10952, #2094, #10290, #2634, #3400, #10122, #9449, #5075, #5294, #6010, #8454, #1002, #6953, #6841, #2684, #6782, #3460, #5133, #1906, #3516, #2568, #890, #10235, #10342, #7682 ),
 ( #5236, #2509, #220, #4466, #116, #6729, #9395, #1793, #7799, #5183, #946, #4239, #8563, #8682, #4349, #57, #8623, #4414, #5896, #173, #1056, #7737, #6905, #6060, #7848, #8511, #9281, #2736, #4293, #1674, #1843, #7625, #5953, #835, #1011, #3569, #6110, #9506, #10178, #9342, #1737 ),
 ( #4677, #10397, #5344, #7166, #10459, #8730, #1110, #6273, #8843, #6224, #8779, #1229, #9562, #2959, #3675, #1284, #6173, #9611, #4626, #8113, #2010, #3785, #2853, #10562, #5396, #1962, #2796, #3618, #9668, #5563, #8895, #1166, #6390, #5454, #434, #4514, #279, #7900, #8055, #4569, #2064 ),
 ( #10618, #7956, #7069, #3012, #8010, #333, #2171, #382, #3728, #7116, #3837, #6332, #9779, #9726, #10512, #2124, #2904, #5511, #7006, #7221, #8944, #1335, #4735, #2223, #5770, #704, #595, #7436, #540, #8213, #9890, #6649, #8270, #7326, #5672, #3991, #4105, #1442, #9212, #1606, #8325 ) ),
 .UNSPECIFIED., .T., .F., .F. ) 
 B_SPLINE_SURFACE_WITH_KNOTS ( ( 4, 3, 4 ),
 ( 3, 2, 2, 2, 2, 2, 2, 2, 2, 2, 2, 2, 2, 2, 2, 2, 2, 2, 2, 2, 3 ),
 ( 0.000000000000000000, 0.5000000000000000000, 1.000000000000000000 ),
 ( 0.000000000000000000, 0.04166666666666666435, 0.08333333333333332871, 0.1250000000000000000, 0.1666666666666666574, 0.2083333333333333426, 0.2500000000000000000, 0.2916666666666666852, 0.3333333333333333148, 0.3750000000000000000, 0.4166666666666666852, 0.4583333333333333148, 0.5000000000000000000, 0.5416666666666666297, 0.5833333333333333703, 0.6250000000000000000, 0.6666666666666666297, 0.7083333333333333703, 0.7500000000000000000, 0.7916666666666666297, 0.8001047462599640836 ),
 .UNSPECIFIED. ) 
 GEOMETRIC_REPRESENTATION_ITEM ( )  RATIONAL_B_SPLINE_SURFACE ( (
 ( 1.000000000000000000, 0.9238795325112867385, 1.000000000000000000, 0.9238795325112867385, 1.000000000000000000, 0.9238795325112867385, 1.000000000000000000, 0.9238795325112867385, 1.000000000000000000, 0.9238795325112867385, 1.000000000000000000, 0.9238795325112867385, 1.000000000000000000, 0.9238795325112867385, 1.000000000000000000, 0.9238795325112867385, 1.000000000000000000, 0.9238795325112867385, 1.000000000000000000, 0.9238795325112867385, 1.000000000000000000, 0.9238795325112867385, 1.000000000000000000, 0.9238795325112867385, 1.000000000000000000, 0.9238795325112867385, 1.000000000000000000, 0.9238795325112867385, 1.000000000000000000, 0.9238795325112867385, 1.000000000000000000, 0.9238795325112867385, 1.000000000000000000, 0.9238795325112867385, 1.000000000000000000, 0.9238795325112867385, 1.000000000000000000, 0.9238795325112867385, 1.000000000000000000, 0.9845845464796294522, 0.9754127805002987817),
 ( 0.3333333333333333703, 0.3079598441704289313, 0.3333333333333333703, 0.3079598441704289313, 0.3333333333333333703, 0.3079598441704289313, 0.3333333333333333703, 0.3079598441704289313, 0.3333333333333333703, 0.3079598441704289313, 0.3333333333333333703, 0.3079598441704289313, 0.3333333333333333703, 0.3079598441704289313, 0.3333333333333333703, 0.3079598441704289313, 0.3333333333333333703, 0.3079598441704289313, 0.3333333333333333703, 0.3079598441704289313, 0.3333333333333333703, 0.3079598441704289313, 0.3333333333333333703, 0.3079598441704289313, 0.3333333333333333703, 0.3079598441704289313, 0.3333333333333333703, 0.3079598441704289313, 0.3333333333333333703, 0.3079598441704289313, 0.3333333333333333703, 0.3079598441704289313, 0.3333333333333333703, 0.3079598441704289313, 0.3333333333333333703, 0.3079598441704289313, 0.3333333333333333703, 0.3079598441704289313, 0.3333333333333333703, 0.3281948488265432062, 0.3251375935000996309),
 ( 0.3333333333333333703, 0.3079598441704289313, 0.3333333333333333703, 0.3079598441704289313, 0.3333333333333333703, 0.3079598441704289313, 0.3333333333333333703, 0.3079598441704289313, 0.3333333333333333703, 0.3079598441704289313, 0.3333333333333333703, 0.3079598441704289313, 0.3333333333333333703, 0.3079598441704289313, 0.3333333333333333703, 0.3079598441704289313, 0.3333333333333333703, 0.3079598441704289313, 0.3333333333333333703, 0.3079598441704289313, 0.3333333333333333703, 0.3079598441704289313, 0.3333333333333333703, 0.3079598441704289313, 0.3333333333333333703, 0.3079598441704289313, 0.3333333333333333703, 0.3079598441704289313, 0.3333333333333333703, 0.3079598441704289313, 0.3333333333333333703, 0.3079598441704289313, 0.3333333333333333703, 0.3079598441704289313, 0.3333333333333333703, 0.3079598441704289313, 0.3333333333333333703, 0.3079598441704289313, 0.3333333333333333703, 0.3281948488265432062, 0.3251375935000996309),
 ( 1.000000000000000000, 0.9238795325112867385, 1.000000000000000000, 0.9238795325112867385, 1.000000000000000000, 0.9238795325112867385, 1.000000000000000000, 0.9238795325112867385, 1.000000000000000000, 0.9238795325112867385, 1.000000000000000000, 0.9238795325112867385, 1.000000000000000000, 0.9238795325112867385, 1.000000000000000000, 0.9238795325112867385, 1.000000000000000000, 0.9238795325112867385, 1.000000000000000000, 0.9238795325112867385, 1.000000000000000000, 0.9238795325112867385, 1.000000000000000000, 0.9238795325112867385, 1.000000000000000000, 0.9238795325112867385, 1.000000000000000000, 0.9238795325112867385, 1.000000000000000000, 0.9238795325112867385, 1.000000000000000000, 0.9238795325112867385, 1.000000000000000000, 0.9238795325112867385, 1.000000000000000000, 0.9238795325112867385, 1.000000000000000000, 0.9238795325112867385, 1.000000000000000000, 0.9845845464796294522, 0.9754127805002987817),
 ( 0.3333333333333333703, 0.3079598441704289313, 0.3333333333333333703, 0.3079598441704289313, 0.3333333333333333703, 0.3079598441704289313, 0.3333333333333333703, 0.3079598441704289313, 0.3333333333333333703, 0.3079598441704289313, 0.3333333333333333703, 0.3079598441704289313, 0.3333333333333333703, 0.3079598441704289313, 0.3333333333333333703, 0.3079598441704289313, 0.3333333333333333703, 0.3079598441704289313, 0.3333333333333333703, 0.3079598441704289313, 0.3333333333333333703, 0.3079598441704289313, 0.3333333333333333703, 0.3079598441704289313, 0.3333333333333333703, 0.3079598441704289313, 0.3333333333333333703, 0.3079598441704289313, 0.3333333333333333703, 0.3079598441704289313, 0.3333333333333333703, 0.3079598441704289313, 0.3333333333333333703, 0.3079598441704289313, 0.3333333333333333703, 0.3079598441704289313, 0.3333333333333333703, 0.3079598441704289313, 0.3333333333333333703, 0.3281948488265432062, 0.3251375935000996309),
 ( 0.3333333333333333703, 0.3079598441704289313, 0.3333333333333333703, 0.3079598441704289313, 0.3333333333333333703, 0.3079598441704289313, 0.3333333333333333703, 0.3079598441704289313, 0.3333333333333333703, 0.3079598441704289313, 0.3333333333333333703, 0.3079598441704289313, 0.3333333333333333703, 0.3079598441704289313, 0.3333333333333333703, 0.3079598441704289313, 0.3333333333333333703, 0.3079598441704289313, 0.3333333333333333703, 0.3079598441704289313, 0.3333333333333333703, 0.3079598441704289313, 0.3333333333333333703, 0.3079598441704289313, 0.3333333333333333703, 0.3079598441704289313, 0.3333333333333333703, 0.3079598441704289313, 0.3333333333333333703, 0.3079598441704289313, 0.3333333333333333703, 0.3079598441704289313, 0.3333333333333333703, 0.3079598441704289313, 0.3333333333333333703, 0.3079598441704289313, 0.3333333333333333703, 0.3079598441704289313, 0.3333333333333333703, 0.3281948488265432062, 0.3251375935000996309),
 ( 1.000000000000000000, 0.9238795325112867385, 1.000000000000000000, 0.9238795325112867385, 1.000000000000000000, 0.9238795325112867385, 1.000000000000000000, 0.9238795325112867385, 1.000000000000000000, 0.9238795325112867385, 1.000000000000000000, 0.9238795325112867385, 1.000000000000000000, 0.9238795325112867385, 1.000000000000000000, 0.9238795325112867385, 1.000000000000000000, 0.9238795325112867385, 1.000000000000000000, 0.9238795325112867385, 1.000000000000000000, 0.9238795325112867385, 1.000000000000000000, 0.9238795325112867385, 1.000000000000000000, 0.9238795325112867385, 1.000000000000000000, 0.9238795325112867385, 1.000000000000000000, 0.9238795325112867385, 1.000000000000000000, 0.9238795325112867385, 1.000000000000000000, 0.9238795325112867385, 1.000000000000000000, 0.9238795325112867385, 1.000000000000000000, 0.9238795325112867385, 1.000000000000000000, 0.9845845464796294522, 0.9754127805002987817) ) ) 
 REPRESENTATION_ITEM ( '' )  SURFACE ( )  );
#4994=CARTESIAN_POINT ( 'NONE',  ( 22.03595509826854126, 19.06622527062933870, 12.00579112326941988 ) ) ;
#5005=CARTESIAN_POINT ( 'NONE',  ( 22.78377297911024257, 19.69285065907503807, 11.00732503135576401 ) ) ;
#5006=( NAMED_UNIT ( * ) PLANE_ANGLE_UNIT ( ) SI_UNIT ( $, .RADIAN. ) );
#5010=CARTESIAN_POINT ( 'NONE',  ( 15.64372318925989802, 17.89181071667436385, 12.19867189564230969 ) ) ;
#5018=CARTESIAN_POINT ( 'NONE',  ( 3.500000000000007994, 28.55025253169416644, 14.51562500000000355 ) ) ;
#5021=CARTESIAN_POINT ( 'NONE',  ( 17.07425424873056130, 16.47910233548095604, 13.06769463237219320 ) ) ;
#5023=CARTESIAN_POINT ( 'NONE',  ( 19.36223501247343393, 16.11237126175916501, 11.95718771041564210 ) ) ;
#5027=CARTESIAN_POINT ( 'NONE',  ( 0.9693646802875628410, 32.52740819067395961, 15.08031658473306891 ) ) ;
#5042=CARTESIAN_POINT ( 'NONE',  ( -1.035533905932736420, 27.49999999999998934, 14.20312500000000355 ) ) ;
#5060=CARTESIAN_POINT ( 'NONE',  ( 22.26413902940654665, 19.29239618210221607, 11.00732503135576401 ) ) ;
#5066=CARTESIAN_POINT ( 'NONE',  ( 19.72987285752124720, 16.32873191470754648, 10.95281372472358861 ) ) ;
#5075=CARTESIAN_POINT ( 'NONE',  ( -3.500000000000002220, 28.55025253169416288, 15.29687500000000178 ) ) ;
#5078=CARTESIAN_POINT ( 'NONE',  ( 16.47160909572790999, 17.06392481020577279, 13.12322671172946897 ) ) ;
#5083=CARTESIAN_POINT ( 'NONE',  ( -2.500000000000005773, 29.99999999999999645, 13.96875000000000355 ) ) ;
#5092=CARTESIAN_POINT ( 'NONE',  ( 19.05040816462259556, 17.06282649731835122, 12.00984920396035172 ) ) ;
#5093=CARTESIAN_POINT ( 'NONE',  ( 1.767766952966372429, 31.76776695296637598, 14.75000000000000355 ) ) ;
#5119=CARTESIAN_POINT ( 'NONE',  ( 20.43380676890320657, 22.25420293214091316, 12.00579112326941988 ) ) ;
#5124=CARTESIAN_POINT ( 'NONE',  ( 22.86591953417209666, 18.42728137938113875, 11.95042449705224819 ) ) ;
#5133=CARTESIAN_POINT ( 'NONE',  ( 1.449747468305833120, 33.50000000000000000, 16.07812500000000355 ) ) ;
#5135=CARTESIAN_POINT ( 'NONE',  ( 15.69051189741946573, 17.84502200851479614, 13.19648031090924789 ) ) ;
#5139=CARTESIAN_POINT ( 'NONE',  ( 19.77604874367146692, 21.01153129092389094, 12.00579112326941988 ) ) ;
#5142=LINE ( 'NONE', #8522, #7206 ) ;
#5150=CARTESIAN_POINT ( 'NONE',  ( 20.17304365239387565, 21.99495017005343200, 12.00579112326981068 ) ) ;
#5151=CARTESIAN_POINT ( 'NONE',  ( 1.035533905932737975, 32.50000000000000711, 16.07812500000000355 ) ) ;
#5175=CARTESIAN_POINT ( 'NONE',  ( 18.86745781575159242, 21.66267592685425569, 11.95042449705185561 ) ) ;
#5176=CARTESIAN_POINT ( 'NONE',  ( 3.500000000000005773, 31.44974746830583001, 15.92187500000000178 ) ) ;
#5183=CARTESIAN_POINT ( 'NONE',  ( -1.383578242660655100, 26.47259180932604039, 13.20531658473306713 ) ) ;
#5185=ADVANCED_FACE ( 'NONE', ( #9534 ), #8651, .F. ) ;
#5186=CARTESIAN_POINT ( 'NONE',  ( 19.75845051886964043, 23.09045650430892849, 12.94889058896590583 ) ) ;
#5187=CARTESIAN_POINT ( 'NONE',  ( 18.07012887690021330, 16.02595819568259827, 12.00212024154935975 ) ) ;
#5188=CARTESIAN_POINT ( 'NONE',  ( 19.13264607096459002, 17.09257730534942965, 12.00833071292064425 ) ) ;
#5190=CARTESIAN_POINT ( 'NONE',  ( -2.458860273309268152, 29.54350846364475203, 15.50141270685246830 ) ) ;
#5197=CARTESIAN_POINT ( 'NONE',  ( 17.79249663040192431, 17.21067465782413919, 12.06642298039558980 ) ) ;
#5201=PRODUCT_DEFINITION_SHAPE ( 'NONE', 'NONE',  #8986 ) ;
#5210=ADVANCED_FACE ( 'NONE', ( #3648 ), #4925, .T. ) ;
#5212=CARTESIAN_POINT ( 'NONE',  ( 2.500000000000008438, 30.00000000000000711, 14.59375000000000178 ) ) ;
#5225=CARTESIAN_POINT ( 'NONE',  ( 21.90605485701305000, 18.97586566459109392, 12.00579112326941988 ) ) ;
#5229=CARTESIAN_POINT ( 'NONE',  ( 15.59693448110033032, 17.93859942483392800, 11.20086348037537327 ) ) ;
#5236=CARTESIAN_POINT ( 'NONE',  ( 2.428085025993350410, 32.52166244231248271, 12.50219158473306358 ) ) ;
#5239=CARTESIAN_POINT ( 'NONE',  ( 24.03139851132786831, 19.63770821034670533, 11.95042449705224996 ) ) ;
#5241=CARTESIAN_POINT ( 'NONE',  ( 24.09141472773967507, 22.06251279622207306, 11.95042449705264076 ) ) ;
#5245=CARTESIAN_POINT ( 'NONE',  ( 2.500000000000008438, 30.00000000000000711, 15.84375000000000355 ) ) ;
#5265=CARTESIAN_POINT ( 'NONE',  ( 1.035533905932737975, 32.50000000000000711, 16.07812500000000355 ) ) ;
#5266=CARTESIAN_POINT ( 'NONE',  ( -1.767766952966370209, 28.23223304703362402, 14.12500000000000355 ) ) ;
#5271=MANIFOLD_SOLID_BREP ( 'Sweep2', #2214 ) ;
#5284=CARTESIAN_POINT ( 'NONE',  ( 19.46525898981753855, 16.20608772750926718, 10.95621100456342312 ) ) ;
#5294=CARTESIAN_POINT ( 'NONE',  ( -2.474873734152916338, 27.52512626584707789, 15.37500000000000355 ) ) ;
#5296=CARTESIAN_POINT ( 'NONE',  ( 18.64799062861727563, 15.97503555906617123, 11.97707131907271005 ) ) ;
#5301=CARTESIAN_POINT ( 'NONE',  ( 16.11564427137601285, 18.83410319690818824, 12.22072830420661660 ) ) ;
#5318=VERTEX_POINT ( 'NONE', #8062 ) ;
#5320=CARTESIAN_POINT ( 'NONE',  ( 1.767766952966377314, 28.23223304703363112, 15.68750000000000355 ) ) ;
#5321=CARTESIAN_POINT ( 'NONE',  ( -2.385244779468109755E-15, 32.50000000000000711, 13.65625000000000355 ) ) ;
#5336=CARTESIAN_POINT ( 'NONE',  ( 21.48473758187327931, 18.75023854587115935, 11.00732503135576401 ) ) ;
#5344=CARTESIAN_POINT ( 'NONE',  ( -0.06616922564517727090, 32.50000000000000711, 12.65844158473306535 ) ) ;
#5346=CARTESIAN_POINT ( 'NONE',  ( 19.34072721801214456, 22.67515267995686656, 12.94889058896629663 ) ) ;
#5349=CARTESIAN_POINT ( 'NONE',  ( 23.22881793621964874, 18.67973499377871960, 11.95042449705234588 ) ) ;
#5350=CARTESIAN_POINT ( 'NONE',  ( 20.08745147943499987, 17.71083118005251933, 12.00579112326941988 ) ) ;
#5358=CARTESIAN_POINT ( 'NONE',  ( 17.36588923991300604, 17.58385822839129986, 12.10347664333366247 ) ) ;
#5366=CARTESIAN_POINT ( 'NONE',  ( -1.449747468305836229, 33.50000000000000000, 13.73437500000000533 ) ) ;
#5370=CARTESIAN_POINT ( 'NONE',  ( -2.500000000000007550, 31.03553390593274486, 16.39062500000000355 ) ) ;
#5371=CARTESIAN_POINT ( 'NONE',  ( 2.500000000000010214, 28.96446609406726225, 14.51562500000000355 ) ) ;
#5381=ORIENTED_EDGE ( 'NONE', *, *, #6748, .T. ) ;
#5388=CARTESIAN_POINT ( 'NONE',  ( 23.28338686706186778, 20.94194386221399640, 11.00732503135556861 ) ) ;
#5396=CARTESIAN_POINT ( 'NONE',  ( -1.720978244806803170, 28.18544433887405987, 14.37719158473306713 ) ) ;
#5398=CARTESIAN_POINT ( 'NONE',  ( 21.82671760412675610, 17.70440453107251244, 11.95042449705224819 ) ) ;
#5402=CARTESIAN_POINT ( 'NONE',  ( 23.89484671925281845, 19.39402032390267649, 11.95042449705224819 ) ) ;
#5404=CARTESIAN_POINT ( 'NONE',  ( 21.28817020210873423, 18.47861593500339694, 13.00425721518307576 ) ) ;
#5422=CARTESIAN_POINT ( 'NONE',  ( -1.734723475976807094E-15, 33.50000000000000000, 14.90625000000000355 ) ) ;
#5427=CARTESIAN_POINT ( 'NONE',  ( 1.814555661125939467, 31.72097824480680828, 15.74780841526694175 ) ) ;
#5428=CARTESIAN_POINT ( 'NONE',  ( 2.500000000000008438, 30.00000000000000711, 14.59375000000000178 ) ) ;
#5430=CARTESIAN_POINT ( 'NONE',  ( 23.33980466280999977, 20.94445964013513617, 12.00579112326902909 ) ) ;
#5447=CARTESIAN_POINT ( 'NONE',  ( 24.26768760078471487, 20.42249838054411271, 10.95195840513859586 ) ) ;
#5454=CARTESIAN_POINT ( 'NONE',  ( 0.9693646802875628410, 32.52740819067395961, 15.08031658473306891 ) ) ;
#5456=CARTESIAN_POINT ( 'NONE',  ( 17.34774915531493278, 16.33073436721105054, 11.04457336562047765 ) ) ;
#5459=CARTESIAN_POINT ( 'NONE',  ( 19.78966864679935611, 21.38900865752197689, 13.00425721518248956 ) ) ;
#5470=CARTESIAN_POINT ( 'NONE',  ( 17.64011212484924940, 17.30965061758477219, 13.07995645546588825 ) ) ;
#5481=CARTESIAN_POINT ( 'NONE',  ( -3.500000000000003109, 29.99999999999999645, 13.96875000000000355 ) ) ;
#5487=CARTESIAN_POINT ( 'NONE',  ( -2.428085025993355295, 32.52166244231248271, 14.81030841526694175 ) ) ;
#5489=DIRECTION ( 'NONE',  ( -0.1561119869140000782, 0.9855205127846302648, -0.06616922564517753458 ) ) ;
#5505=CARTESIAN_POINT ( 'NONE',  ( 19.82941471729559524, 23.00258574805652856, 10.95195840513859231 ) ) ;
#5511=CARTESIAN_POINT ( 'NONE',  ( 1.035533905932737975, 32.50000000000000711, 14.82812500000000178 ) ) ;
#5514=CARTESIAN_POINT ( 'NONE',  ( 15.59693448110033032, 17.93859942483392800, 11.20086348037537327 ) ) ;
#5517=CARTESIAN_POINT ( 'NONE',  ( 21.41520517525563605, 22.70178780811528441, 13.00425721518307753 ) ) ;
#5524=CARTESIAN_POINT ( 'NONE',  ( 20.43380676890320657, 22.25420293214091316, 12.00579112326941988 ) ) ;
#5532=CARTESIAN_POINT ( 'NONE',  ( 0.06616922564517314920, 33.50000000000000000, 17.15405841526694175 ) ) ;
#5538=CARTESIAN_POINT ( 'NONE',  ( 3.472591809326051937, 28.48408330604899419, 15.51343341526694353 ) ) ;
#5556=CARTESIAN_POINT ( 'NONE',  ( 18.58376669197321007, 17.02366754649298031, 11.02344032946268548 ) ) ;
#5563=CARTESIAN_POINT ( 'NONE',  ( 2.527408190673965382, 29.03063531971243449, 14.76781658473306535 ) ) ;
#5566=CARTESIAN_POINT ( 'NONE',  ( 16.06885556321644160, 18.88089190506775594, 11.22291988893967840 ) ) ;
#5571=CARTESIAN_POINT ( 'NONE',  ( 16.08167231043895384, 17.45386159549338245, 13.15979613361243494 ) ) ;
#5577=CARTESIAN_POINT ( 'NONE',  ( 19.95755123817951215, 17.62047157401400810, 12.00579112326941988 ) ) ;
#5583=CARTESIAN_POINT ( 'NONE',  ( 2.521662442312485819, 32.42808502599335441, 16.99780841526693820 ) ) ;
#5588=CARTESIAN_POINT ( 'NONE',  ( -2.505208318772514708, 29.86938897312880314, 17.48140433884295319 ) ) ;
#5612=CARTESIAN_POINT ( 'NONE',  ( 20.05551109708751412, 20.00475302350064766, 11.00732503135517426 ) ) ;
#5622=CARTESIAN_POINT ( 'NONE',  ( 22.42093126068789033, 23.47289781856171587, 10.95195840513859231 ) ) ;
#5624=CARTESIAN_POINT ( 'NONE',  ( 15.69051189741946573, 17.84502200851479614, 13.19648031090924789 ) ) ;
#5630=PRODUCT_DEFINITION_FORMATION_WITH_SPECIFIED_SOURCE ( 'ANY', '', #10340, .NOT_KNOWN. ) ;
#5632=CARTESIAN_POINT ( 'NONE',  ( 21.41951502703731691, 22.64547864373410135, 12.00579112326941988 ) ) ;
#5640=CARTESIAN_POINT ( 'NONE',  ( -1.101703131577916883, 32.47259180932605460, 12.73656658473306358 ) ) ;
#5647=CARTESIAN_POINT ( 'NONE',  ( -2.472591809326051937, 31.10170313157791000, 16.13843341526694530 ) ) ;
#5649=CARTESIAN_POINT ( 'NONE',  ( 16.89796509758633647, 18.05178237071871195, 12.14735994959122856 ) ) ;
#5663=CARTESIAN_POINT ( 'NONE',  ( 20.46928886811658188, 22.21026755401432240, 11.00732503135576401 ) ) ;
#5672=CARTESIAN_POINT ( 'NONE',  ( -2.385244779468109755E-15, 32.50000000000000711, 16.15625000000000355 ) ) ;
#5674=CARTESIAN_POINT ( 'NONE',  ( 16.98270770525814299, 16.57081904430127395, 11.07189675232624104 ) ) ;
#5676=CARTESIAN_POINT ( 'NONE',  ( 17.02848097699435215, 16.52496068989110967, 12.06979569234921890 ) ) ;
#5682=CARTESIAN_POINT ( 'NONE',  ( -2.500000000000007550, 30.06616922564517580, 17.46655841526694175 ) ) ;
#5686=CARTESIAN_POINT ( 'NONE',  ( 20.11906803080876571, 17.66537948065741759, 13.00425721518307576 ) ) ;
#5687=CARTESIAN_POINT ( 'NONE',  ( 16.58601566935801586, 18.36373179894819074, 12.17661548709639696 ) ) ;
#5690=CARTESIAN_POINT ( 'NONE',  ( 1.383578242660657098, 33.52740819067396671, 15.08031658473306891 ) ) ;
#5691=CARTESIAN_POINT ( 'NONE',  ( 16.23246227876473213, 18.01017840835489991, 12.17661548709639696 ) ) ;
#5695=CARTESIAN_POINT ( 'NONE',  ( 0.06616922564517249694, 32.50000000000000711, 15.90405841526694175 ) ) ;
#5705=CARTESIAN_POINT ( 'NONE',  ( 3.500000000000005773, 31.44974746830583001, 14.67187500000000178 ) ) ;
#5710=CARTESIAN_POINT ( 'NONE',  ( 22.93505243896877133, 21.90805399618153970, 11.00732503135576401 ) ) ;
#5722=CARTESIAN_POINT ( 'NONE',  ( 20.05551109708751412, 20.00475302350064766, 11.00732503135517426 ) ) ;
#5727=CARTESIAN_POINT ( 'NONE',  ( 19.90085419568980640, 16.36478119802090703, 11.95042571680015442 ) ) ;
#5731=CARTESIAN_POINT ( 'NONE',  ( -2.474873734152916338, 27.52512626584707789, 14.12500000000000355 ) ) ;
#5733=CARTESIAN_POINT ( 'NONE',  ( 23.94195266346560658, 19.36439822498074648, 12.94889058896590583 ) ) ;
#5739=CARTESIAN_POINT ( 'NONE',  ( 3.472591809326047052, 31.51591669395100936, 14.92406658473306713 ) ) ;
#5744=CARTESIAN_POINT ( 'NONE',  ( -1.101703131577911776, 27.52740819067395250, 16.45093341526693820 ) ) ;
#5754=CARTESIAN_POINT ( 'NONE',  ( -1.734723475976807094E-15, 33.50000000000000000, 14.90625000000000355 ) ) ;
#5761=CARTESIAN_POINT ( 'NONE',  ( 16.35082997044643704, 18.59891749786092063, 12.19867189564230969 ) ) ;
#5770=CARTESIAN_POINT ( 'NONE',  ( -1.767766952966370209, 28.23223304703362402, 15.37500000000000355 ) ) ;
#5773=CARTESIAN_POINT ( 'NONE',  ( 18.58376669197321007, 17.02366754649298031, 11.02344032946268548 ) ) ;
#5776=DIRECTION ( 'NONE',  ( 0.9876851083892502770, 0.1564548710207356030, 0.000000000000000000 ) ) ;
#5777=CARTESIAN_POINT ( 'NONE',  ( 22.50783536177859645, 18.11075086187001659, 12.94889058896590583 ) ) ;
#5783=CARTESIAN_POINT ( 'NONE',  ( -2.472591809326051937, 31.10170313157791000, 17.38843341526693820 ) ) ;
#5786=CARTESIAN_POINT ( 'NONE',  ( 18.11095311068464397, 15.98247068297658835, 13.00034071860445550 ) ) ;
#5790=CARTESIAN_POINT ( 'NONE',  ( -2.521662442312484931, 32.42808502599334730, 14.06469158473306358 ) ) ;
#5802=CARTESIAN_POINT ( 'NONE',  ( 18.27511531525127353, 17.01097670698189290, 12.03680973694848966 ) ) ;
#5811=CIRCLE ( 'NONE', #5985, 0.4999999999999985567 ) ;
#5812=CARTESIAN_POINT ( 'NONE',  ( 3.500000000000005329, 30.00000000000000000, 14.59375000000000178 ) ) ;
#5821=CARTESIAN_POINT ( 'NONE',  ( 20.08745147943499987, 17.71083118005251933, 12.00579112326941988 ) ) ;
#5828=CARTESIAN_POINT ( 'NONE',  ( 15.92569759632967497, 17.60983630960342339, 13.17442390236345418 ) ) ;
#5833=CARTESIAN_POINT ( 'NONE',  ( 18.23429108146684641, 17.05446421968790460, 11.03858925989339390 ) ) ;
#5836=CARTESIAN_POINT ( 'NONE',  ( 16.42482038756834228, 17.11071351836534049, 12.12541829646253078 ) ) ;
#5843=CARTESIAN_POINT ( 'NONE',  ( -1.449747468305836229, 33.50000000000000000, 13.73437500000000533 ) ) ;
#5845=CARTESIAN_POINT ( 'NONE',  ( 16.77403034288735029, 16.76147925670542094, 13.09486341078152805 ) ) ;
#5846=CARTESIAN_POINT ( 'NONE',  ( 21.82671760412675610, 17.70440453107251244, 11.95042449705224819 ) ) ;
#5850=CARTESIAN_POINT ( 'NONE',  ( -1.814555661125939912, 31.72097824480680117, 15.31469158473306713 ) ) ;
#5858=CARTESIAN_POINT ( 'NONE',  ( 2.474873734152918558, 32.47487373415292211, 13.50000000000000355 ) ) ;
#5860=CARTESIAN_POINT ( 'NONE',  ( 4.553649124439118623E-15, 27.49999999999999289, 14.28125000000000355 ) ) ;
#5868=CARTESIAN_POINT ( 'NONE',  ( -1.035533905932742638, 32.50000000000000000, 13.73437500000000533 ) ) ;
#5873=DIRECTION ( 'NONE',  ( -0.7055570967602625698, 0.7055570967602455834, 0.06616922564518108729 ) ) ;
#5885=CARTESIAN_POINT ( 'NONE',  ( 17.74785087444460885, 17.25574343990722070, 11.06843699004799397 ) ) ;
#5888=CARTESIAN_POINT ( 'NONE',  ( 20.75790788474667181, 23.61206934513595357, 12.94889058896590583 ) ) ;
#5896=CARTESIAN_POINT ( 'NONE',  ( -0.06616922564517661864, 33.50000000000000000, 13.90844158473306713 ) ) ;
#5900=CARTESIAN_POINT ( 'NONE',  ( 20.18549546789347460, 16.49528347911771675, 12.94888893485705061 ) ) ;
#5905=CARTESIAN_POINT ( 'NONE',  ( -2.500000000000007550, 31.03553390593274486, 15.14062500000000355 ) ) ;
#5913=CARTESIAN_POINT ( 'NONE',  ( 23.31827848602400621, 20.57738196266585362, 12.00579112326941988 ) ) ;
#5914=CARTESIAN_POINT ( 'NONE',  ( -1.767766952966375094, 31.76776695296636888, 15.06250000000000355 ) ) ;
#5938=CARTESIAN_POINT ( 'NONE',  ( 21.42382487881899777, 22.58916947935290764, 11.00732503135576401 ) ) ;
#5944=CARTESIAN_POINT ( 'NONE',  ( 22.47621881040483771, 18.15620256126511478, 11.95042449705224819 ) ) ;
#5953=CARTESIAN_POINT ( 'NONE',  ( 2.428085025993350410, 32.52166244231248271, 15.00219158473306535 ) ) ;
#5956=CARTESIAN_POINT ( 'NONE',  ( 17.43584335925693196, 16.24128823292743817, 13.04062965360331106 ) ) ;
#5958=CARTESIAN_POINT ( 'NONE',  ( 18.79784185921769790, 16.99560944861731215, 12.01584860934582366 ) ) ;
#5961=CARTESIAN_POINT ( 'NONE',  ( 1.767766952966372429, 31.76776695296637598, 16.00000000000000355 ) ) ;
#5971=CARTESIAN_POINT ( 'NONE',  ( 23.13231036272843966, 20.08340223762181154, 12.00579112326941988 ) ) ;
#5972=CARTESIAN_POINT ( 'NONE',  ( -2.500000000000005773, 29.99999999999999645, 15.21875000000000355 ) ) ;
#5985=AXIS2_PLACEMENT_3D ( 'NONE', #6177, #7959, #7120 ) ;
#5998=AXIS2_PLACEMENT_3D ( 'NONE', #6922, #10311, #140 ) ;
#6001=CARTESIAN_POINT ( 'NONE',  ( 23.34652552892808330, 18.77429515943753202, 11.95042449705224819 ) ) ;
#6002=CARTESIAN_POINT ( 'NONE',  ( -1.734723475976807094E-15, 33.50000000000000000, 16.15625000000000355 ) ) ;
#6010=CARTESIAN_POINT ( 'NONE',  ( -1.449747468305830678, 26.49999999999999289, 15.45312500000000178 ) ) ;
#6012=CARTESIAN_POINT ( 'NONE',  ( 16.42482038756834228, 17.11071351836534049, 12.12541829646253078 ) ) ;
#6015=CARTESIAN_POINT ( 'NONE',  ( 16.42482038756834228, 17.11071351836534049, 12.12541829646253078 ) ) ;
#6016=CARTESIAN_POINT ( 'NONE',  ( 19.84380896203909828, 21.37294244821887546, 12.00579112326902731 ) ) ;
#6018=CARTESIAN_POINT ( 'NONE',  ( -2.500000000000007550, 31.03553390593274486, 13.89062500000000355 ) ) ;
#6028=CARTESIAN_POINT ( 'NONE',  ( -1.035533905932742860, 32.50000000000000000, 16.23437500000000355 ) ) ;
#6052=CARTESIAN_POINT ( 'NONE',  ( 19.79393261808261428, 23.04652112618272852, 11.95042449705224819 ) ) ;
#6060=CARTESIAN_POINT ( 'NONE',  ( -3.472591809326043499, 28.48408330604899064, 14.29906658473306358 ) ) ;
#6062=CARTESIAN_POINT ( 'NONE',  ( 20.77365933115271446, 23.55783661745384094, 11.95042449705224819 ) ) ;
#6065=CARTESIAN_POINT ( 'NONE',  ( 15.92724728075741680, 19.02250018754875072, 13.24059312800850030 ) ) ;
#6067=CARTESIAN_POINT ( 'NONE',  ( -2.385244779468109755E-15, 32.50000000000000711, 14.90625000000000355 ) ) ;
#6075=CARTESIAN_POINT ( 'NONE',  ( 19.13264607096459002, 17.09257730534942965, 12.00833071292064425 ) ) ;
#6077=CARTESIAN_POINT ( 'NONE',  ( 19.55162244606592381, 17.33808635661342024, 12.00579012602852735 ) ) ;
#6087=CARTESIAN_POINT ( 'NONE',  ( 2.527408190673967159, 30.96936468028756906, 16.91968341526693820 ) ) ;
#6102=CARTESIAN_POINT ( 'NONE',  ( 22.08651808663882932, 17.88512374315008557, 11.95042449705224819 ) ) ;
#6110=CARTESIAN_POINT ( 'NONE',  ( -2.521662442312484931, 32.42808502599334730, 15.31469158473306713 ) ) ;
#6113=CARTESIAN_POINT ( 'NONE',  ( 22.60611905166032898, 18.24656216730335601, 11.95042449705224819 ) ) ;
#6116=CARTESIAN_POINT ( 'NONE',  ( 22.43871220627207563, 23.52649944903870249, 11.95042449705224819 ) ) ;
#6117=CARTESIAN_POINT ( 'NONE',  ( 16.74199038346592872, 18.20775708483950694, 12.16198771834549497 ) ) ;
#6121=( NAMED_UNIT ( * ) PLANE_ANGLE_UNIT ( ) SI_UNIT ( $, .RADIAN. ) );
#6143=CARTESIAN_POINT ( 'NONE',  ( -2.527408190673963162, 29.03063531971243094, 16.29468341526694530 ) ) ;
#6144=CARTESIAN_POINT ( 'NONE',  ( -2.500000000000007550, 31.03553390593274486, 16.39062500000000355 ) ) ;
#6163=CARTESIAN_POINT ( 'NONE',  ( 18.02930464311577907, 16.06944570838860642, 11.00389976449426399 ) ) ;
#6173=CARTESIAN_POINT ( 'NONE',  ( 1.720978244806805169, 31.81455566112594013, 13.75219158473306535 ) ) ;
#6175=CARTESIAN_POINT ( 'NONE',  ( 18.81331750051067075, 21.67874213615617762, 12.94889058896551326 ) ) ;
#6177=CARTESIAN_POINT ( 'NONE',  ( 2.121320343559645494, 32.12132034355964549, 13.50000000000000355 ) ) ;
#6193=CARTESIAN_POINT ( 'NONE',  ( 3.903127820947815962E-15, 26.49999999999999289, 14.28125000000000355 ) ) ;
#6197=CARTESIAN_POINT ( 'NONE',  ( 1.101703131577913553, 32.47259180932605460, 14.57593341526694175 ) ) ;
#6198=CARTESIAN_POINT ( 'NONE',  ( -1.767766952966375094, 31.76776695296636888, 13.81250000000000355 ) ) ;
#6217=CARTESIAN_POINT ( 'NONE',  ( 18.23429108146684641, 17.05446421968790460, 11.03858925989339390 ) ) ;
#6224=CARTESIAN_POINT ( 'NONE',  ( -0.9693646802875608426, 27.47259180932603684, 13.20531658473306713 ) ) ;
#6226=CARTESIAN_POINT ( 'NONE',  ( 16.50280774463635680, 17.03272616129868666, 12.11810441208646338 ) ) ;
#6228=CARTESIAN_POINT ( 'NONE',  ( 16.54959645279592451, 16.98593745313911896, 13.11591282735340336 ) ) ;
#6243=CARTESIAN_POINT ( 'NONE',  ( 2.428085025993357071, 27.47833755768751374, 16.68530841526694175 ) ) ;
#6247=CARTESIAN_POINT ( 'NONE',  ( 2.500000000000007550, 31.03553390593274486, 15.92187500000000178 ) ) ;
#6248=CARTESIAN_POINT ( 'NONE',  ( 1.035533905932743970, 27.49999999999999289, 14.35937500000000711 ) ) ;
#6250=CARTESIAN_POINT ( 'NONE',  ( 22.29575558078030895, 19.24694448270711788, 12.00579112326941988 ) ) ;
#6265=CARTESIAN_POINT ( 'NONE',  ( 23.98154255942039370, 19.66242269470938453, 10.95195840513859586 ) ) ;
#6273=CARTESIAN_POINT ( 'NONE',  ( -2.472591809326046608, 28.89829686842208289, 13.04906658473306891 ) ) ;
#6275=CARTESIAN_POINT ( 'NONE',  ( 18.76105380172462844, 21.09515122317004909, 11.95042449705224819 ) ) ;
#6279=CARTESIAN_POINT ( 'NONE',  ( 22.32737213215407479, 19.20149278331202325, 13.00425721518307576 ) ) ;
#6289=CARTESIAN_POINT ( 'NONE',  ( 19.85760542366876535, 20.31250532737884384, 12.00579112326941988 ) ) ;
#6299=CARTESIAN_POINT ( 'NONE',  ( 1.449747468305836673, 26.49999999999999289, 14.35937500000000711 ) ) ;
#6307=CARTESIAN_POINT ( 'NONE',  ( -2.385244779468109755E-15, 32.50000000000000711, 16.15625000000000355 ) ) ;
#6308=CARTESIAN_POINT ( 'NONE',  ( 1.035533905932737975, 32.50000000000000711, 13.57812500000000178 ) ) ;
#6310=CARTESIAN_POINT ( 'NONE',  ( 19.95755123817951215, 17.62047157401400810, 12.00579112326941988 ) ) ;
#6326=CARTESIAN_POINT ( 'NONE',  ( 22.93674656822681612, 23.24041807713223307, 10.95195840513859231 ) ) ;
#6331=VERTEX_POINT ( 'NONE', #4065 ) ;
#6332=CARTESIAN_POINT ( 'NONE',  ( 1.035533905932743970, 27.49999999999999289, 14.35937500000000711 ) ) ;
#6335=CARTESIAN_POINT ( 'NONE',  ( 21.01569960522067504, 17.20769859423666048, 10.95195840513859231 ) ) ;
#6341=CARTESIAN_POINT ( 'NONE',  ( 22.86397682584157565, 19.61629903322988966, 13.00425721518307753 ) ) ;
#6349=CARTESIAN_POINT ( 'NONE',  ( 23.13231036272843966, 20.08340223762181154, 12.00579112326941988 ) ) ;
#6358=CARTESIAN_POINT ( 'NONE',  ( 23.89484671925281845, 19.39402032390267649, 11.95042449705224819 ) ) ;
#6363=CARTESIAN_POINT ( 'NONE',  ( 3.500000000000007994, 28.55025253169416644, 15.76562500000000178 ) ) ;
#6367=CARTESIAN_POINT ( 'NONE',  ( -3.505208318772512488, 29.79067687212226545, 17.48140433884295319 ) ) ;
#6369=CARTESIAN_POINT ( 'NONE',  ( -0.06616922564517119243, 26.49999999999999289, 15.27905841526694175 ) ) ;
#6384=CARTESIAN_POINT ( 'NONE',  ( 17.08513846059531005, 17.86460900771146143, 11.12760988119559258 ) ) ;
#6390=CARTESIAN_POINT ( 'NONE',  ( 1.720978244806805169, 31.81455566112594013, 15.00219158473306535 ) ) ;
#6392=CARTESIAN_POINT ( 'NONE',  ( 16.14406960823794179, 17.39146429769401081, 11.14955153432450530 ) ) ;
#6394=CARTESIAN_POINT ( 'NONE',  ( 20.19688095354152324, 19.67517542290917731, 13.00425721518307753 ) ) ;
#6400=CARTESIAN_POINT ( 'NONE',  ( 17.83714238635922911, 17.16560587574106123, 13.06440897074317853 ) ) ;
#6405=CARTESIAN_POINT ( 'NONE',  ( 3.500000000000005329, 30.00000000000000000, 15.84375000000000355 ) ) ;
#6411=CARTESIAN_POINT ( 'NONE',  ( 0.06616922564517314920, 33.50000000000000000, 15.90405841526694175 ) ) ;
#6428=CARTESIAN_POINT ( 'NONE',  ( 17.45361707773674809, 17.49611573659335662, 12.09524845743996657 ) ) ;
#6438=CARTESIAN_POINT ( 'NONE',  ( 16.85117638942448082, 18.09857107888056760, 11.14955153432450530 ) ) ;
#6440=CARTESIAN_POINT ( 'NONE',  ( 16.23764702455707720, 17.29788688137487185, 13.14516836485838169 ) ) ;
#6446=CARTESIAN_POINT ( 'NONE',  ( 22.63806431670481700, 19.48506897666907989, 12.00579112326951758 ) ) ;
#6452=CARTESIAN_POINT ( 'NONE',  ( -2.472591809326046608, 28.89829686842208289, 13.04906658473306891 ) ) ;
#6458=CARTESIAN_POINT ( 'NONE',  ( 2.527408190673967159, 30.96936468028756906, 15.66968341526694175 ) ) ;
#6480=CARTESIAN_POINT ( 'NONE',  ( 22.10027471249113162, 22.50626116107413921, 11.00732503135576401 ) ) ;
#6492=CARTESIAN_POINT ( 'NONE',  ( 15.36174878203077476, 18.17378512388119915, 11.22291988893967840 ) ) ;
#6495=CARTESIAN_POINT ( 'NONE',  ( 16.90694777372845437, 16.62861179130368683, 12.08020438729360180 ) ) ;
#6501=ORIENTED_EDGE ( 'NONE', *, *, #10765, .T. ) ;
#6502=CARTESIAN_POINT ( 'NONE',  ( 16.78877909162549642, 18.16096837667994279, 13.15979613361243494 ) ) ;
#6508=CARTESIAN_POINT ( 'NONE',  ( -2.527408190673963162, 30.96936468028755840, 14.14281658473306713 ) ) ;
#6514=CARTESIAN_POINT ( 'NONE',  ( 1.101703131577913553, 32.47259180932605460, 14.57593341526694175 ) ) ;
#6527=CARTESIAN_POINT ( 'NONE',  ( 3.500000000000007550, 28.55025253169416644, 14.51562500000000355 ) ) ;
#6536=CARTESIAN_POINT ( 'NONE',  ( 19.89794927727885110, 21.35687623891577758, 11.00732503135556861 ) ) ;
#6543=DIRECTION ( 'NONE',  ( 0.9876851083892502770, 0.1564548710207356030, 0.000000000000000000 ) ) ;
#6549=CARTESIAN_POINT ( 'NONE',  ( 19.91130943667480224, 20.32997460694367575, 11.00732503135576401 ) ) ;
#6552=CARTESIAN_POINT ( 'NONE',  ( 19.39692024064573062, 16.06847318657456469, 12.95562166920678138 ) ) ;
#6557=CARTESIAN_POINT ( 'NONE',  ( -1.734723475976807094E-15, 33.50000000000000000, 13.65625000000000355 ) ) ;
#6559=CARTESIAN_POINT ( 'NONE',  ( 21.93767140838681584, 18.93041396519599928, 13.00425721518307576 ) ) ;
#6563=CARTESIAN_POINT ( 'NONE',  ( -0.9693646802875608426, 27.47259180932603684, 14.45531658473306535 ) ) ;
#6568=CARTESIAN_POINT ( 'NONE',  ( -2.500000000000007550, 30.06616922564517580, 17.46655841526694175 ) ) ;
#6577=CARTESIAN_POINT ( 'NONE',  ( -3.500000000000003997, 31.44974746830583001, 15.14062500000000355 ) ) ;
#6581=CARTESIAN_POINT ( 'NONE',  ( 22.42490604353609029, 22.35994869845890065, 11.00732503135576401 ) ) ;
#6593=CARTESIAN_POINT ( 'NONE',  ( 23.28338686706186778, 20.94194386221399640, 11.00732503135556861 ) ) ;
#6599=CARTESIAN_POINT ( 'NONE',  ( 24.14247934234231963, 22.08663129433533001, 12.94889058896630019 ) ) ;
#6604=CARTESIAN_POINT ( 'NONE',  ( -3.472591809326048384, 31.51591669395100936, 16.13843341526694530 ) ) ;
#6606=CARTESIAN_POINT ( 'NONE',  ( 16.95349311633468403, 16.58206632678699677, 13.07803561935715742 ) ) ;
#6611=CARTESIAN_POINT ( 'NONE',  ( -0.9693646802875608426, 27.47259180932603684, 13.20531658473306713 ) ) ;
#6612=CARTESIAN_POINT ( 'NONE',  ( 16.58601566935801586, 18.36373179894819074, 12.17661548709639696 ) ) ;
#6630=CARTESIAN_POINT ( 'NONE',  ( 2.474873734152918558, 32.47487373415292211, 13.50000000000000355 ) ) ;
#6640=CARTESIAN_POINT ( 'NONE',  ( 20.43380676890320657, 22.25420293214091316, 12.00579112326941988 ) ) ;
#6649=CARTESIAN_POINT ( 'NONE',  ( 2.500000000000007550, 31.03553390593274486, 15.92187500000000178 ) ) ;
#6653=CARTESIAN_POINT ( 'NONE',  ( 20.46928886811658188, 22.21026755401432240, 11.00732503135576401 ) ) ;
#6659=CARTESIAN_POINT ( 'NONE',  ( 18.83541841558448837, 19.97999999654625825, 12.94889058896590583 ) ) ;
#6668=CARTESIAN_POINT ( 'NONE',  ( -3.472591809326048384, 31.51591669395100936, 17.38843341526693820 ) ) ;
#6671=CARTESIAN_POINT ( 'NONE',  ( 21.33873319047917150, 17.29751440752404434, 12.94889058896590583 ) ) ;
#6678=CARTESIAN_POINT ( 'NONE',  ( -1.383578242660655100, 26.47259180932604039, 13.20531658473306713 ) ) ;
#6698=AXIS2_PLACEMENT_3D ( 'NONE', #7004, #3616, #9504 ) ;
#6704=STYLED_ITEM ( 'NONE', ( #598 ), #7322 ) ;
#6719=CARTESIAN_POINT ( 'NONE',  ( 22.84119893477061680, 19.75612935582806529, 11.00732503135576401 ) ) ;
#6722=CARTESIAN_POINT ( 'NONE',  ( 17.31044041986821469, 16.31370680995936695, 13.04945978079559765 ) ) ;
#6729=CARTESIAN_POINT ( 'NONE',  ( -3.527408190673960053, 31.38357824266065066, 12.89281658473306535 ) ) ;
#6731=CARTESIAN_POINT ( 'NONE',  ( 19.39692024064573062, 16.06847318657456469, 12.95562166920678138 ) ) ;
#6735=CARTESIAN_POINT ( 'NONE',  ( 4.553649124439118623E-15, 27.49999999999999289, 14.28125000000000355 ) ) ;
#6743=CARTESIAN_POINT ( 'NONE',  ( 21.05771646464872404, 22.57981893131178452, 12.00579112326941988 ) ) ;
#6748=EDGE_CURVE ( 'NONE', #7325, #8937, #10072, .T. ) ;
#6769=CARTESIAN_POINT ( 'NONE',  ( 19.09861202765586086, 17.13671095651997689, 11.00988473025352121 ) ) ;
#6773=CARTESIAN_POINT ( 'NONE',  ( 20.62599888145302529, 16.93661977612163128, 10.95195840513859231 ) ) ;
#6782=CARTESIAN_POINT ( 'NONE',  ( 3.500000000000005773, 31.44974746830583356, 15.92187500000000178 ) ) ;
#6785=CARTESIAN_POINT ( 'NONE',  ( 23.09245737654782360, 19.89859478643763069, 13.00425721518307753 ) ) ;
#6786=CARTESIAN_POINT ( 'NONE',  ( 16.19085831639981166, 17.34467558953214095, 12.14735994959122856 ) ) ;
#6787=CARTESIAN_POINT ( 'NONE',  ( 23.13231036272843966, 20.08340223762181154, 12.00579112326941988 ) ) ;
#6789=CARTESIAN_POINT ( 'NONE',  ( 4.553649124439118623E-15, 27.49999999999999289, 15.53125000000000355 ) ) ;
#6798=CARTESIAN_POINT ( 'NONE',  ( 18.62184541094303114, 16.98042197548449295, 12.02177981800743112 ) ) ;
#6807=EDGE_CURVE ( 'NONE', #5318, #2956, #3651, .T. ) ;
#6833=CARTESIAN_POINT ( 'NONE',  ( 20.15426471261298147, 16.54100339847095213, 11.95042283504686154 ) ) ;
#6841=CARTESIAN_POINT ( 'NONE',  ( 3.500000000000007994, 28.55025253169416644, 15.76562500000000178 ) ) ;
#6844=CARTESIAN_POINT ( 'NONE',  ( 16.03488360227938969, 17.50065030365295016, 12.16198771834549497 ) ) ;
#6847=CARTESIAN_POINT ( 'NONE',  ( 23.31827848602400621, 20.57738196266585362, 12.00579112326941988 ) ) ;
#6850=CARTESIAN_POINT ( 'NONE',  ( 2.500000000000007550, 31.03553390593274486, 15.92187500000000178 ) ) ;
#6854=EDGE_CURVE ( 'NONE', #9431, #6331, #4177, .T. ) ;
#6855=ORIENTED_EDGE ( 'NONE', *, *, #10765, .F. ) ;
#6867=CARTESIAN_POINT ( 'NONE',  ( 1.767766952966372429, 31.76776695296637598, 13.50000000000000355 ) ) ;
#6888=CARTESIAN_POINT ( 'NONE',  ( 19.55162244606592381, 17.33808635661342024, 12.00579012602852735 ) ) ;
#6894=CARTESIAN_POINT ( 'NONE',  ( 23.22881793621964874, 18.67973499377871960, 11.95042449705234588 ) ) ;
#6905=CARTESIAN_POINT ( 'NONE',  ( -3.500000000000001332, 29.93383077435482065, 14.22094158473306535 ) ) ;
#6907=CARTESIAN_POINT ( 'NONE',  ( 18.83541841558448837, 19.97999999654625825, 12.94889058896590583 ) ) ;
#6908=CARTESIAN_POINT ( 'NONE',  ( 20.26791470906062997, 16.62008925861079334, 11.95042449705224819 ) ) ;
#6909=CARTESIAN_POINT ( 'NONE',  ( 22.69616945897178084, 19.53356342368596898, 12.00579112326941988 ) ) ;
#6916=CARTESIAN_POINT ( 'NONE',  ( 18.79784185921769790, 16.99560944861731215, 12.01584860934582366 ) ) ;
#6918=CARTESIAN_POINT ( 'NONE',  ( 22.11805565807571128, 22.55986279155152374, 12.00579112326941988 ) ) ;
#6922=CARTESIAN_POINT ( 'NONE',  ( 19.86292016999849608, 19.38279280778333202, 11.97810781016083403 ) ) ;
#6928=CARTESIAN_POINT ( 'NONE',  ( -0.9693646802875689472, 32.52740819067395961, 17.23218341526694530 ) ) ;
#6929=CARTESIAN_POINT ( 'NONE',  ( -1.767766952966375094, 31.76776695296636888, 15.06250000000000355 ) ) ;
#6944=CARTESIAN_POINT ( 'NONE',  ( 18.90462188152790901, 16.04371289204410189, 10.96879988954262153 ) ) ;
#6953=CARTESIAN_POINT ( 'NONE',  ( 2.474873734152922111, 27.52512626584708144, 15.68750000000000355 ) ) ;
#6955=CARTESIAN_POINT ( 'NONE',  ( 16.65878245872646701, 16.87675144720473952, 12.10347664333366247 ) ) ;
#6956=CARTESIAN_POINT ( 'NONE',  ( 0.000000000000000000, 0.000000000000000000, 0.000000000000000000 ) ) ;
#6959=CARTESIAN_POINT ( 'NONE',  ( 23.33980466280999977, 20.94445964013513617, 12.00579112326902909 ) ) ;
#6981=CARTESIAN_POINT ( 'NONE',  ( -1.035533905932736420, 27.49999999999998934, 15.45312500000000178 ) ) ;
#6982=CARTESIAN_POINT ( 'NONE',  ( 1.767766952966377314, 28.23223304703363112, 15.68750000000000355 ) ) ;
#6998=CARTESIAN_POINT ( 'NONE',  ( 18.76105380172462844, 21.09515122317004909, 11.95042449705224819 ) ) ;
#7000=CARTESIAN_POINT ( 'NONE',  ( -3.500000000000003997, 31.44974746830583001, 16.39062500000000355 ) ) ;
#7004=CARTESIAN_POINT ( 'NONE',  ( 2.121320343559645494, 32.12132034355964549, 13.50000000000000355 ) ) ;
#7006=CARTESIAN_POINT ( 'NONE',  ( -2.385244779468109755E-15, 32.50000000000000711, 14.90625000000000355 ) ) ;
#7011=CARTESIAN_POINT ( 'NONE',  ( 24.32342464814431438, 20.41340561598360992, 11.95042449705224996 ) ) ;
#7014=CARTESIAN_POINT ( 'NONE',  ( 17.45361707773674809, 17.49611573659335662, 12.09524845743996657 ) ) ;
#7024=EDGE_CURVE ( 'NONE', #10270, #2599, #7252, .T. ) ;
#7028=CARTESIAN_POINT ( 'NONE',  ( 16.89796509758404852, 18.05178237072099989, 12.14735994959144350 ) ) ;
#7036=CARTESIAN_POINT ( 'NONE',  ( -1.734723475976807094E-15, 33.50000000000000000, 13.65625000000000355 ) ) ;
#7042=CARTESIAN_POINT ( 'NONE',  ( 2.472591809326055046, 28.89829686842209355, 15.51343341526694353 ) ) ;
#7043=CARTESIAN_POINT ( 'NONE',  ( -2.500000000000004885, 29.80321974748363090, 16.48359592357600434 ) ) ;
#7051=CARTESIAN_POINT ( 'NONE',  ( -2.963055325167751164, 29.53063538693776735, 16.49922112211940117 ) ) ;
#7060=CARTESIAN_POINT ( 'NONE',  ( 15.83366986443827962, 19.11607760386789323, 11.24497629747462568 ) ) ;
#7069=CARTESIAN_POINT ( 'NONE',  ( -2.385244779468109755E-15, 32.50000000000000711, 13.65625000000000355 ) ) ;
#7071=CARTESIAN_POINT ( 'NONE',  ( 15.64372318925989802, 17.89181071667436385, 12.19867189564230969 ) ) ;
#7075=CARTESIAN_POINT ( 'NONE',  ( 19.80390141066272491, 20.29503604781401904, 13.00425721518307753 ) ) ;
#7088=CARTESIAN_POINT ( 'NONE',  ( 1.449747468305833120, 33.50000000000000000, 13.57812500000000178 ) ) ;
#7092=CARTESIAN_POINT ( 'NONE',  ( 2.500000000000009770, 29.93383077435482420, 15.59155841526693997 ) ) ;
#7093=CARTESIAN_POINT ( 'NONE',  ( -2.500000000000007550, 31.03553390593274486, 13.89062500000000355 ) ) ;
#7094=CARTESIAN_POINT ( 'NONE',  ( 19.85760542366876535, 20.31250532737884384, 12.00579112326941988 ) ) ;
#7110=CARTESIAN_POINT ( 'NONE',  ( 17.54702143963720928, 17.40274154661815587, 11.08429399133878057 ) ) ;
#7113=EDGE_LOOP ( 'NONE', ( #4126, #2126 ) ) ;
#7116=CARTESIAN_POINT ( 'NONE',  ( -1.035533905932736420, 27.49999999999998934, 14.20312500000000355 ) ) ;
#7118=CARTESIAN_POINT ( 'NONE',  ( 22.44460225903107187, 18.20165426066020942, 10.95195840513859231 ) ) ;
#7120=DIRECTION ( 'NONE',  ( -0.7071067811865479058, -0.7071067811865470176, 0.000000000000000000 ) ) ;
#7121=CARTESIAN_POINT ( 'NONE',  ( 19.72936730704260810, 17.39430066254168139, 13.00425721518307576 ) ) ;
#7129=FACE_OUTER_BOUND ( 'NONE', #971, .T. ) ;
#7136=CARTESIAN_POINT ( 'NONE',  ( -3.500000000000003553, 31.44974746830583356, 15.14062500000000355 ) ) ;
#7140=CARTESIAN_POINT ( 'NONE',  ( 1.720978244806812496, 28.18544433887406342, 16.68530841526694175 ) ) ;
#7143=CARTESIAN_POINT ( 'NONE',  ( 22.11805565807571128, 22.55986279155152374, 12.00579112326941988 ) ) ;
#7159=CARTESIAN_POINT ( 'NONE',  ( 19.09861202765586086, 17.13671095651997689, 11.00988473025352121 ) ) ;
#7166=CARTESIAN_POINT ( 'NONE',  ( -1.101703131577916883, 32.47259180932605460, 12.73656658473306358 ) ) ;
#7168=CARTESIAN_POINT ( 'NONE',  ( 17.22114890795359798, 16.40384437412513208, 11.05348780010051435 ) ) ;
#7172=CARTESIAN_POINT ( 'NONE',  ( 21.34179237787287065, 23.66094220255952152, 11.95042449705224819 ) ) ;
#7173=CARTESIAN_POINT ( 'NONE',  ( 18.65992412991285221, 16.93717640447601269, 13.02011930655217675 ) ) ;
#7181=CARTESIAN_POINT ( 'NONE',  ( 19.58285320134683261, 17.29236643726018130, 13.00425622583864715 ) ) ;
#7192=CARTESIAN_POINT ( 'NONE',  ( -2.474873734152916338, 27.52512626584707789, 15.37500000000000355 ) ) ;
#7197=CARTESIAN_POINT ( 'NONE',  ( -1.515916693951006478, 26.52740819067394895, 15.20093341526694353 ) ) ;
#7198=CARTESIAN_POINT ( 'NONE',  ( 3.500000000000007994, 29.93383077435482420, 15.59155841526693997 ) ) ;
#7200=CARTESIAN_POINT ( 'NONE',  ( 22.03595509826854126, 19.06622527062933870, 12.00579112326941988 ) ) ;
#7206=VECTOR ( 'NONE', #4301, 999.9999999999998863 ) ;
#7215=CARTESIAN_POINT ( 'NONE',  ( 20.70533613433985920, 18.20808090964021986, 11.00732503135576401 ) ) ;
#7221=CARTESIAN_POINT ( 'NONE',  ( -1.035533905932742638, 32.50000000000000000, 14.98437500000000711 ) ) ;
#7224=CARTESIAN_POINT ( 'NONE',  ( 22.05490153526506703, 17.93057544254518376, 10.95195840513859231 ) ) ;
#7229=CARTESIAN_POINT ( 'NONE',  ( 19.98916778955327800, 17.57501987461890991, 13.00425721518307576 ) ) ;
#7236=CARTESIAN_POINT ( 'NONE',  ( 17.41267794807257374, 17.53706952023173216, 13.10128505860060066 ) ) ;
#7244=CARTESIAN_POINT ( 'NONE',  ( -3.500000000000002665, 29.72450764647708255, 16.48359592357600434 ) ) ;
#7250=CARTESIAN_POINT ( 'NONE',  ( 2.500000000000009770, 29.93383077435482420, 16.84155841526694175 ) ) ;
#7252=( BOUNDED_CURVE ( )  B_SPLINE_CURVE ( 3, ( #2611, #2548, #5828, #3441 ),
 .UNSPECIFIED., .F., .F. ) 
 B_SPLINE_CURVE_WITH_KNOTS ( ( 4, 4 ),
 ( 3.469446951953614189E-18, 0.001563228649568143037 ),
 .UNSPECIFIED. ) 
 CURVE ( )  GEOMETRIC_REPRESENTATION_ITEM ( )  RATIONAL_B_SPLINE_CURVE ( ( 1.000000000000000000, 0.3333333333333327597, 0.3333333333333334814, 1.000000000000000666 ) ) 
 REPRESENTATION_ITEM ( '' )  );
#7253=CARTESIAN_POINT ( 'NONE',  ( 19.86292016999849608, 19.38279280778333202, 11.97810781016083403 ) ) ;
#7267=CARTESIAN_POINT ( 'NONE',  ( 22.41005638895160601, 19.39388128063383476, 11.00732503135576401 ) ) ;
#7271=CARTESIAN_POINT ( 'NONE',  ( -2.963055325167751164, 29.53063538693776735, 16.49922112211940117 ) ) ;
#7277=CARTESIAN_POINT ( 'NONE',  ( 16.86040243112223180, 16.67515725582037689, 11.08237315523004973 ) ) ;
#7279=CARTESIAN_POINT ( 'NONE',  ( 22.67082259973814828, 19.44041185113230341, 13.00425721518326938 ) ) ;
#7286=CARTESIAN_POINT ( 'NONE',  ( 22.44007493706583745, 19.34731747087121434, 12.00579112326928133 ) ) ;
#7292=CARTESIAN_POINT ( 'NONE',  ( 3.500000000000003997, 30.06616922564517580, 14.84594158473306713 ) ) ;
#7300=CARTESIAN_POINT ( 'NONE',  ( 2.500000000000009770, 29.93383077435482420, 15.59155841526693997 ) ) ;
#7303=CARTESIAN_POINT ( 'NONE',  ( -2.385244779468109755E-15, 32.50000000000000711, 13.65625000000000355 ) ) ;
#7318=CARTESIAN_POINT ( 'NONE',  ( 23.13231036272843966, 20.08340223762181154, 12.00579112326941988 ) ) ;
#7322=ADVANCED_BREP_SHAPE_REPRESENTATION ( '', ( #5271, #308 ), #3340 ) ;
#7325=VERTEX_POINT ( 'NONE', #3927 ) ;
#7326=CARTESIAN_POINT ( 'NONE',  ( 1.035533905932737975, 32.50000000000000711, 16.07812500000000355 ) ) ;
#7328=CARTESIAN_POINT ( 'NONE',  ( 20.49609864019753402, 16.84626017008312360, 10.95195840513859231 ) ) ;
#7331=CARTESIAN_POINT ( 'NONE',  ( 16.50280774463635680, 17.03272616129868666, 12.11810441208646338 ) ) ;
#7338=CARTESIAN_POINT ( 'NONE',  ( 21.25655365073496839, 18.52406763439849513, 12.00579112326941988 ) ) ;
#7345=CARTESIAN_POINT ( 'NONE',  ( -2.521662442312484931, 32.42808502599334730, 15.31469158473306713 ) ) ;
#7352=CARTESIAN_POINT ( 'NONE',  ( -2.428085025993355295, 32.52166244231248271, 14.81030841526694175 ) ) ;
#7375=CARTESIAN_POINT ( 'NONE',  ( 19.77604874367146692, 21.01153129092389094, 12.00579112326941988 ) ) ;
#7386=CARTESIAN_POINT ( 'NONE',  ( 19.89794927727885110, 21.35687623891577758, 11.00732503135556861 ) ) ;
#7388=CARTESIAN_POINT ( 'NONE',  ( 19.36223501247343393, 16.11237126175916501, 11.95718771041564210 ) ) ;
#7394=CARTESIAN_POINT ( 'NONE',  ( 1.383578242660662871, 26.47259180932604039, 16.60718341526694175 ) ) ;
#7396=CARTESIAN_POINT ( 'NONE',  ( 22.69616945897178084, 19.53356342368596898, 12.00579112326941988 ) ) ;
#7402=CARTESIAN_POINT ( 'NONE',  ( 0.06616922564517879746, 26.50000000000000000, 14.53344158473306535 ) ) ;
#7408=CARTESIAN_POINT ( 'NONE',  ( -3.527408190673961386, 28.61642175733934224, 15.04468341526694175 ) ) ;
#7411=CARTESIAN_POINT ( 'NONE',  ( 17.59356678224322934, 17.35619608210146581, 12.08212522340233264 ) ) ;
#7421=CARTESIAN_POINT ( 'NONE',  ( 3.903127820947815962E-15, 26.49999999999999289, 14.28125000000000355 ) ) ;
#7427=CARTESIAN_POINT ( 'NONE',  ( 22.69616945897178084, 19.53356342368596898, 12.00579112326941988 ) ) ;
#7436=CARTESIAN_POINT ( 'NONE',  ( 1.035533905932743970, 27.49999999999999289, 15.60937500000000711 ) ) ;
#7439=CARTESIAN_POINT ( 'NONE',  ( 19.01572293645009637, 17.10672457250295508, 11.01141524516921422 ) ) ;
#7440=FILL_AREA_STYLE_COLOUR ( '', #2453 ) ;
#7444=CARTESIAN_POINT ( 'NONE',  ( 23.26157621925297647, 18.63507786824203549, 12.94889058896600353 ) ) ;
#7451=CARTESIAN_POINT ( 'NONE',  ( 0.06616922564517314920, 33.50000000000000000, 14.65405841526694353 ) ) ;
#7453=CARTESIAN_POINT ( 'NONE',  ( 22.06757164964230711, 19.02077357123424406, 13.00425721518307576 ) ) ;
#7458=CARTESIAN_POINT ( 'NONE',  ( 1.515916693951011140, 26.52740819067395250, 14.61156658473306713 ) ) ;
#7459=CARTESIAN_POINT ( 'NONE',  ( 15.83212018001054133, 17.70341372592255524, 11.17880707182957778 ) ) ;
#7476=CARTESIAN_POINT ( 'NONE',  ( -2.500000000000007550, 31.03553390593274486, 13.89062500000000355 ) ) ;
#7482=CARTESIAN_POINT ( 'NONE',  ( 22.11805565807571128, 22.55986279155152374, 12.00579112326941988 ) ) ;
#7485=ORIENTED_EDGE ( 'NONE', *, *, #3909, .T. ) ;
#7494=CARTESIAN_POINT ( 'NONE',  ( 17.45361707773674809, 17.49611573659335662, 12.09524845743996657 ) ) ;
#7498=CARTESIAN_POINT ( 'NONE',  ( 15.17335179141131185, 18.36218211452176519, 12.24278471274156388 ) ) ;
#7505=CARTESIAN_POINT ( 'NONE',  ( 0.06616922564517314920, 33.50000000000000000, 15.90405841526694175 ) ) ;
#7508=ADVANCED_FACE ( 'NONE', ( #10866 ), #4989, .T. ) ;
#7509=CARTESIAN_POINT ( 'NONE',  ( 20.68923198420054987, 16.84571637733143490, 12.94889058896590583 ) ) ;
#7513=CARTESIAN_POINT ( 'NONE',  ( -1.720978244806803170, 28.18544433887405987, 14.37719158473306713 ) ) ;
#7539=CARTESIAN_POINT ( 'NONE',  ( 22.82387490247590733, 19.65457484615246386, 12.00579112326941988 ) ) ;
#7553=CARTESIAN_POINT ( 'NONE',  ( 17.86810043078960319, 17.16701444005803268, 12.06109941161078325 ) ) ;
#7558=CARTESIAN_POINT ( 'NONE',  ( 17.39179625728592882, 16.28601130006924791, 12.04260150961189524 ) ) ;
#7564=CARTESIAN_POINT ( 'NONE',  ( 3.500000000000005773, 31.44974746830583356, 14.67187500000000178 ) ) ;
#7567=CARTESIAN_POINT ( 'NONE',  ( 22.13583660366028738, 22.61346442202890472, 13.00425721518307753 ) ) ;
#7570=CARTESIAN_POINT ( 'NONE',  ( 16.50280774463635680, 17.03272616129868666, 12.11810441208646338 ) ) ;
#7573=CARTESIAN_POINT ( 'NONE',  ( 2.527408190673965382, 29.03063531971243449, 14.76781658473306535 ) ) ;
#7585=CARTESIAN_POINT ( 'NONE',  ( 18.79784185921769790, 16.99560944861731215, 12.01584860934582366 ) ) ;
#7600=( GEOMETRIC_REPRESENTATION_CONTEXT ( 3 ) GLOBAL_UNCERTAINTY_ASSIGNED_CONTEXT ( ( #8970 ) ) GLOBAL_UNIT_ASSIGNED_CONTEXT ( ( #9737, #6121, #9570 ) ) REPRESENTATION_CONTEXT ( 'NONE', 'WORKASPACE' ) );
#7613=CARTESIAN_POINT ( 'NONE',  ( 22.66010611969070965, 19.57566612754892432, 11.00732503135576401 ) ) ;
#7618=CARTESIAN_POINT ( 'NONE',  ( 23.64018263364375017, 19.06693133664117212, 11.95042449705224819 ) ) ;
#7625=CARTESIAN_POINT ( 'NONE',  ( 3.472591809326047052, 31.51591669395100936, 14.92406658473306713 ) ) ;
#7628=CARTESIAN_POINT ( 'NONE',  ( 22.89753608554585540, 18.38182967998604056, 12.94889058896590583 ) ) ;
#7629=CARTESIAN_POINT ( 'NONE',  ( 17.02848097699435215, 16.52496068989110967, 12.06979569234921890 ) ) ;
#7632=CARTESIAN_POINT ( 'NONE',  ( -1.767766952966370209, 28.23223304703362402, 14.12500000000000355 ) ) ;
#7642=CARTESIAN_POINT ( 'NONE',  ( 19.13264607096459002, 17.09257730534942965, 12.00833071292064425 ) ) ;
#7643=CARTESIAN_POINT ( 'NONE',  ( -2.500000000000005773, 29.99999999999999645, 16.46875000000000355 ) ) ;
#7669=CARTESIAN_POINT ( 'NONE',  ( 20.17304365239387565, 21.99495017005343200, 12.00579112326981068 ) ) ;
#7673=CARTESIAN_POINT ( 'NONE',  ( 22.44460225903107187, 18.20165426066020942, 10.95195840513859231 ) ) ;
#7682=CARTESIAN_POINT ( 'NONE',  ( -3.456897879362375470, 29.45240795142740353, 16.49922112211940117 ) ) ;
#7684=CARTESIAN_POINT ( 'NONE',  ( 21.30711663910541276, 17.34296610691914253, 11.95042449705224819 ) ) ;
#7685=( BOUNDED_CURVE ( )  B_SPLINE_CURVE ( 2, ( #4135, #3307, #7303, #1369, #8146, #10696, #3088, #2256, #8194, #571, #5860, #9297, #10308, #10088, #1760, #2476, #5093, #8640, #2703, #8473, #5914, #9412, #5972, #8410, #9243, #857, #8532, #10254, #10194, #9362, #1696, #2593, #4258, #5151, #909, #6028, #3365, #1021, #7643, #19, #1860 ),
 .UNSPECIFIED., .F., .T. ) 
 B_SPLINE_CURVE_WITH_KNOTS ( ( 3, 2, 2, 2, 2, 2, 2, 2, 2, 2, 2, 2, 2, 2, 2, 2, 2, 2, 2, 2, 3 ),
 ( 0.000000000000000000, 0.04166666666666666435, 0.08333333333333332871, 0.1250000000000000000, 0.1666666666666666574, 0.2083333333333333148, 0.2500000000000000000, 0.2916666666666666852, 0.3333333333333333148, 0.3750000000000000000, 0.4166666666666666297, 0.4583333333333333148, 0.5000000000000000000, 0.5416666666666666297, 0.5833333333333333703, 0.6250000000000000000, 0.6666666666666666297, 0.7083333333333334814, 0.7500000000000000000, 0.7916666666666666297, 0.8001047462599640836 ),
 .UNSPECIFIED. ) 
 CURVE ( )  GEOMETRIC_REPRESENTATION_ITEM ( )  RATIONAL_B_SPLINE_CURVE ( ( 1.000000000000000000, 0.9238795325112867385, 1.000000000000000000, 0.9238795325112867385, 1.000000000000000000, 0.9238795325112867385, 1.000000000000000000, 0.9238795325112867385, 1.000000000000000000, 0.9238795325112867385, 1.000000000000000000, 0.9238795325112867385, 1.000000000000000000, 0.9238795325112867385, 1.000000000000000000, 0.9238795325112867385, 1.000000000000000000, 0.9238795325112867385, 1.000000000000000000, 0.9238795325112867385, 1.000000000000000000, 0.9238795325112867385, 1.000000000000000000, 0.9238795325112867385, 1.000000000000000000, 0.9238795325112867385, 1.000000000000000000, 0.9238795325112867385, 1.000000000000000000, 0.9238795325112867385, 1.000000000000000000, 0.9238795325112867385, 1.000000000000000000, 0.9238795325112867385, 1.000000000000000000, 0.9238795325112867385, 1.000000000000000000, 0.9238795325112867385, 1.000000000000000000, 0.9845845464796294522, 0.9754127805002987817 ) ) 
 REPRESENTATION_ITEM ( '' )  );
#7687=CARTESIAN_POINT ( 'NONE',  ( 15.87890888817147150, 17.65662501776163040, 12.17661548709639341 ) ) ;
#7688=CARTESIAN_POINT ( 'NONE',  ( 17.13192716875488131, 17.81782029955189728, 12.12541829646253078 ) ) ;
#7691=CARTESIAN_POINT ( 'NONE',  ( 1.035533905932737975, 32.50000000000000711, 14.82812500000000178 ) ) ;
#7724=CARTESIAN_POINT ( 'NONE',  ( 23.31827848602400621, 20.57738196266585362, 12.00579112326941988 ) ) ;
#7729=CARTESIAN_POINT ( 'NONE',  ( 16.37803167940877458, 17.15750222652490820, 11.12760988119559258 ) ) ;
#7730=CARTESIAN_POINT ( 'NONE',  ( 1.449747468305832898, 33.50000000000000000, 16.07812500000000355 ) ) ;
#7737=CARTESIAN_POINT ( 'NONE',  ( -3.527408190673960053, 31.38357824266065066, 14.14281658473306713 ) ) ;
#7741=CARTESIAN_POINT ( 'NONE',  ( 20.65761543282678758, 16.89116807672653664, 11.95042449705224819 ) ) ;
#7744=CARTESIAN_POINT ( 'NONE',  ( 19.76265562249496099, 16.28401831655332543, 11.95127577209155234 ) ) ;
#7746=AXIS2_PLACEMENT_3D ( 'NONE', #5691, #4187, #2348 ) ;
#7764=CARTESIAN_POINT ( 'NONE',  ( 0.06616922564517249694, 32.50000000000000711, 14.65405841526694353 ) ) ;
#7768=CARTESIAN_POINT ( 'NONE',  ( 1.035533905932737975, 32.50000000000000711, 16.07812500000000355 ) ) ;
#7790=CARTESIAN_POINT ( 'NONE',  ( 17.74381166370891449, 16.14600641939347980, 11.01911823137775492 ) ) ;
#7799=CARTESIAN_POINT ( 'NONE',  ( -2.428085025993349078, 27.47833755768751374, 13.12719158473306535 ) ) ;
#7801=CARTESIAN_POINT ( 'NONE',  ( 17.26579466391090634, 16.35877559204224951, 12.05147379044805866 ) ) ;
#7803=CARTESIAN_POINT ( 'NONE',  ( 23.54706165660595829, 18.96431965174070555, 11.95042449705224819 ) ) ;
#7804=CARTESIAN_POINT ( 'NONE',  ( 22.44007493706583745, 19.34731747087121434, 12.00579112326928133 ) ) ;
#7806=CARTESIAN_POINT ( 'NONE',  ( 2.500000000000010214, 28.96446609406726225, 14.51562500000000355 ) ) ;
#7822=CARTESIAN_POINT ( 'NONE',  ( 1.720978244806812496, 28.18544433887406342, 15.43530841526694175 ) ) ;
#7826=CYLINDRICAL_SURFACE ( 'NONE', #389, 0.4999999999999883982 ) ;
#7839=CARTESIAN_POINT ( 'NONE',  ( 20.12303395733248834, 16.58672331782418752, 10.95195673523667246 ) ) ;
#7848=CARTESIAN_POINT ( 'NONE',  ( -2.428085025993349078, 27.47833755768751374, 14.37719158473306713 ) ) ;
#7850=CARTESIAN_POINT ( 'NONE',  ( 22.98142095123195716, 18.50759888342988546, 11.95042449705211141 ) ) ;
#7852=CARTESIAN_POINT ( 'NONE',  ( 24.03139851132786831, 19.63770821034670533, 11.95042449705224996 ) ) ;
#7863=CARTESIAN_POINT ( 'NONE',  ( 16.35082997044643704, 18.59891749786092063, 12.19867189564230969 ) ) ;
#7871=CARTESIAN_POINT ( 'NONE',  ( 2.474873734152918558, 32.47487373415292211, 14.75000000000000355 ) ) ;
#7875=CARTESIAN_POINT ( 'NONE',  ( -0.06616922564517033201, 27.49999999999998934, 15.27905841526694175 ) ) ;
#7876=CARTESIAN_POINT ( 'NONE',  ( 2.500000000000010214, 28.96446609406726225, 15.76562500000000178 ) ) ;
#7892=CARTESIAN_POINT ( 'NONE',  ( 22.84119893477061680, 19.75612935582806529, 11.00732503135576401 ) ) ;
#7900=CARTESIAN_POINT ( 'NONE',  ( -2.527408190673963162, 30.96936468028755840, 15.39281658473306358 ) ) ;
#7904=CARTESIAN_POINT ( 'NONE',  ( 17.02848097699435215, 16.52496068989110967, 12.06979569234921890 ) ) ;
#7907=CARTESIAN_POINT ( 'NONE',  ( 23.79237391907785693, 22.55645663433636017, 11.95042449705224819 ) ) ;
#7908=CARTESIAN_POINT ( 'NONE',  ( 20.12931512496741249, 22.03068688373604900, 13.00425721518366728 ) ) ;
#7919=CARTESIAN_POINT ( 'NONE',  ( 17.59356678224322934, 17.35619608210146581, 12.08212522340233264 ) ) ;
#7927=CARTESIAN_POINT ( 'NONE',  ( -2.521662442312483599, 27.57191497400664204, 16.37280841526694175 ) ) ;
#7931=CARTESIAN_POINT ( 'NONE',  ( -2.472591809326051937, 31.10170313157791000, 14.88843341526694353 ) ) ;
#7933=CARTESIAN_POINT ( 'NONE',  ( 18.62184541094303114, 16.98042197548449295, 12.02177981800743112 ) ) ;
#7949=CARTESIAN_POINT ( 'NONE',  ( 16.85117638942448082, 18.09857107888056760, 11.14955153432450530 ) ) ;
#7956=CARTESIAN_POINT ( 'NONE',  ( 1.035533905932737975, 32.50000000000000711, 13.57812500000000178 ) ) ;
#7958=CARTESIAN_POINT ( 'NONE',  ( 18.60991190964745456, 16.01828113007465504, 10.97873183052796620 ) ) ;
#7959=DIRECTION ( 'NONE',  ( -0.7055570967602537991, 0.7055570967602550203, 0.06616922564517474514 ) ) ;
#7960=MECHANICAL_DESIGN_GEOMETRIC_PRESENTATION_REPRESENTATION('',(#10265),#7600);
#7961=CARTESIAN_POINT ( 'NONE',  ( 16.77403034288735029, 16.76147925670542094, 13.09486341078152805 ) ) ;
#7979=CARTESIAN_POINT ( 'NONE',  ( 1.383578242660657098, 33.52740819067396671, 12.58031658473306713 ) ) ;
#7984=CARTESIAN_POINT ( 'NONE',  ( 0.9693646802875698354, 27.47259180932603684, 16.60718341526694175 ) ) ;
#7985=CARTESIAN_POINT ( 'NONE',  ( -1.035533905932736420, 27.49999999999998934, 15.45312500000000178 ) ) ;
#7986=CARTESIAN_POINT ( 'NONE',  ( 23.13231036272843966, 20.08340223762181154, 12.00579112326941988 ) ) ;
#8004=CARTESIAN_POINT ( 'NONE',  ( 22.60530603367148927, 19.52972610220585636, 11.00732503135576401 ) ) ;
#8010=CARTESIAN_POINT ( 'NONE',  ( -1.767766952966375094, 31.76776695296636888, 13.81250000000000355 ) ) ;
#8012=CARTESIAN_POINT ( 'NONE',  ( 20.12303395733248834, 16.58672331782418752, 10.95195673523667246 ) ) ;
#8015=CARTESIAN_POINT ( 'NONE',  ( 17.64011212484924940, 17.30965061758477219, 13.07995645546588825 ) ) ;
#8022=CARTESIAN_POINT ( 'NONE',  ( 19.77604874367146692, 21.01153129092389094, 12.00579112326941988 ) ) ;
#8029=CARTESIAN_POINT ( 'NONE',  ( -1.449747468305830678, 26.49999999999999289, 14.20312500000000355 ) ) ;
#8033=CARTESIAN_POINT ( 'NONE',  ( 2.428085025993357071, 27.47833755768751374, 16.68530841526694175 ) ) ;
#8034=CARTESIAN_POINT ( 'NONE',  ( -2.500000000000007550, 30.06616922564517580, 14.96655841526694175 ) ) ;
#8036=CARTESIAN_POINT ( 'NONE',  ( 19.13264607096459002, 17.09257730534942965, 12.00833071292064425 ) ) ;
#8049=CARTESIAN_POINT ( 'NONE',  ( 19.92593468680574986, 17.66592327340909918, 11.00732503135576401 ) ) ;
#8055=CARTESIAN_POINT ( 'NONE',  ( -2.500000000000003997, 29.93383077435482065, 15.47094158473306535 ) ) ;
#8057=CARTESIAN_POINT ( 'NONE',  ( 23.98154255942039370, 19.66242269470938453, 10.95195840513859586 ) ) ;
#8061=CARTESIAN_POINT ( 'NONE',  ( 17.91214753276079819, 17.12229137291643610, 13.05912755560225236 ) ) ;
#8062=CARTESIAN_POINT ( 'NONE',  ( -3.456897879362374582, 29.45240795142739998, 16.49922112211940117 ) ) ;
#8070=CARTESIAN_POINT ( 'NONE',  ( 17.25670323398246353, 17.69304423432567930, 13.11591282735340336 ) ) ;
#8081=CARTESIAN_POINT ( 'NONE',  ( -2.474873734152920335, 32.47487373415291501, 16.31250000000000355 ) ) ;
#8088=CARTESIAN_POINT ( 'NONE',  ( 2.521662442312485819, 32.42808502599335441, 14.49780841526694175 ) ) ;
#8105=CARTESIAN_POINT ( 'NONE',  ( 21.22493709936120254, 18.56951933379358621, 11.00732503135576401 ) ) ;
#8109=ORIENTED_EDGE ( 'NONE', *, *, #3959, .T. ) ;
#8113=CARTESIAN_POINT ( 'NONE',  ( -1.101703131577916883, 32.47259180932605460, 13.98656658473306713 ) ) ;
#8116=CARTESIAN_POINT ( 'NONE',  ( 23.50695973324029353, 19.00259546466308791, 10.95195840513859231 ) ) ;
#8119=CARTESIAN_POINT ( 'NONE',  ( 23.39622245855813176, 20.94697541805627239, 13.00425721518248956 ) ) ;
#8129=CARTESIAN_POINT ( 'NONE',  ( 20.73695268571362504, 18.16262921024512167, 12.00579112326941988 ) ) ;
#8136=CARTESIAN_POINT ( 'NONE',  ( 2.521662442312487151, 27.57191497400665270, 14.68969158473306535 ) ) ;
#8142=CARTESIAN_POINT ( 'NONE',  ( -3.472591809326048384, 31.51591669395100936, 16.13843341526694530 ) ) ;
#8146=CARTESIAN_POINT ( 'NONE',  ( -1.767766952966375094, 31.76776695296636888, 13.81250000000000355 ) ) ;
#8159=CARTESIAN_POINT ( 'NONE',  ( 19.13264607096459002, 17.09257730534942965, 12.00833071292064425 ) ) ;
#8167=CARTESIAN_POINT ( 'NONE',  ( 19.72987285752124720, 16.32873191470754648, 10.95281372472358861 ) ) ;
#8171=CARTESIAN_POINT ( 'NONE',  ( 15.40853749019034069, 18.12699641572163145, 12.22072830420661660 ) ) ;
#8177=CARTESIAN_POINT ( 'NONE',  ( 19.84380896203909828, 21.37294244821887546, 12.00579112326902731 ) ) ;
#8185=CARTESIAN_POINT ( 'NONE',  ( 1.101703131577918438, 27.52740819067395606, 13.36156658473306535 ) ) ;
#8191=CARTESIAN_POINT ( 'NONE',  ( -2.500000000000007550, 30.06616922564517580, 16.21655841526694175 ) ) ;
#8194=CARTESIAN_POINT ( 'NONE',  ( -1.767766952966370209, 28.23223304703362402, 14.12500000000000355 ) ) ;
#8205=CARTESIAN_POINT ( 'NONE',  ( 20.47715220320264962, 17.98190999816754498, 12.00579112326941988 ) ) ;
#8213=CARTESIAN_POINT ( 'NONE',  ( 2.500000000000010214, 28.96446609406726225, 15.76562500000000178 ) ) ;
#8215=CARTESIAN_POINT ( 'NONE',  ( 22.93505243896877133, 21.90805399618153970, 11.00732503135576401 ) ) ;
#8217=CARTESIAN_POINT ( 'NONE',  ( 19.53332707643461319, 16.11782042516817981, 12.95310296989756260 ) ) ;
#8222=CARTESIAN_POINT ( 'NONE',  ( -3.527408190673961386, 28.61642175733934224, 16.29468341526694530 ) ) ;
#8224=CARTESIAN_POINT ( 'NONE',  ( 21.28817020210873423, 18.47861593500339694, 13.00425721518307576 ) ) ;
#8230=CARTESIAN_POINT ( 'NONE',  ( 1.101703131577918438, 27.52740819067395606, 14.61156658473306713 ) ) ;
#8239=CARTESIAN_POINT ( 'NONE',  ( 1.515916693951008254, 33.47259180932604750, 14.57593341526694175 ) ) ;
#8253=CARTESIAN_POINT ( 'NONE',  ( 1.449747468305836673, 26.49999999999999289, 15.60937500000000533 ) ) ;
#8261=CARTESIAN_POINT ( 'NONE',  ( 18.27511531525127353, 17.01097670698189290, 12.03680973694848966 ) ) ;
#8270=CARTESIAN_POINT ( 'NONE',  ( 1.767766952966372429, 31.76776695296637598, 16.00000000000000355 ) ) ;
#8273=CARTESIAN_POINT ( 'NONE',  ( 23.08245441082096150, 20.10811672198468969, 11.00732503135576401 ) ) ;
#8276=CARTESIAN_POINT ( 'NONE',  ( 19.34072721801214456, 22.67515267995686656, 12.94889058896629663 ) ) ;
#8282=CARTESIAN_POINT ( 'NONE',  ( 2.474873734152918558, 32.47487373415292211, 13.50000000000000355 ) ) ;
#8284=CARTESIAN_POINT ( 'NONE',  ( 23.02513694122459498, 21.97618599832468433, 13.00425721518307753 ) ) ;
#8290=CARTESIAN_POINT ( 'NONE',  ( 1.720978244806805169, 31.81455566112594013, 13.75219158473306535 ) ) ;
#8309=CARTESIAN_POINT ( 'NONE',  ( 1.449747468305832898, 33.50000000000000000, 13.57812500000000533 ) ) ;
#8314=CARTESIAN_POINT ( 'NONE',  ( 22.98009469009668138, 21.94211999725310491, 12.00579112326941988 ) ) ;
#8325=CARTESIAN_POINT ( 'NONE',  ( -2.469212770973128190, 29.60886282244813117, 16.49922112211940117 ) ) ;
#8328=CARTESIAN_POINT ( 'NONE',  ( 20.28019557727208166, 19.74811736329550982, 11.00732503135576401 ) ) ;
#8331=CARTESIAN_POINT ( 'NONE',  ( 21.33748252609158058, 23.71725136694109892, 12.94889058896590583 ) ) ;
#8337=CARTESIAN_POINT ( 'NONE',  ( -3.500000000000002220, 28.55025253169416288, 14.04687500000000355 ) ) ;
#8340=CARTESIAN_POINT ( 'NONE',  ( 23.38258886820915095, 18.73219245557438484, 12.94889058896590583 ) ) ;
#8342=CARTESIAN_POINT ( 'NONE',  ( 20.65761543282678758, 16.89116807672653664, 11.95042449705224819 ) ) ;
#8345=CARTESIAN_POINT ( 'NONE',  ( 1.383578242660657098, 33.52740819067396671, 13.83031658473306535 ) ) ;
#8354=CARTESIAN_POINT ( 'NONE',  ( 20.00651627240589647, 19.97666299463432438, 12.00579112326824216 ) ) ;
#8362=CARTESIAN_POINT ( 'NONE',  ( 1.035533905932743970, 27.49999999999999289, 14.35937500000000711 ) ) ;
#8367=CARTESIAN_POINT ( 'NONE',  ( 17.65010306112908722, 17.31038946799904465, 12.07741653513508417 ) ) ;
#8381=CARTESIAN_POINT ( 'NONE',  ( 22.99824548812224378, 19.95783898428147651, 11.00732503135576401 ) ) ;
#8385=CARTESIAN_POINT ( 'NONE',  ( 16.72700999897183038, 16.80849948458634557, 12.09707671258119888 ) ) ;
#8393=CARTESIAN_POINT ( 'NONE',  ( -1.449747468305830678, 26.49999999999999289, 14.20312500000000355 ) ) ;
#8395=CARTESIAN_POINT ( 'NONE',  ( 23.22159451225019566, 21.65168511467167889, 13.00425721518366728 ) ) ;
#8399=CARTESIAN_POINT ( 'NONE',  ( -0.06616922564517727090, 32.50000000000000711, 15.15844158473306535 ) ) ;
#8410=CARTESIAN_POINT ( 'NONE',  ( -2.500000000000004441, 28.96446609406725514, 15.29687500000000533 ) ) ;
#8439=CARTESIAN_POINT ( 'NONE',  ( 18.06244887585786074, 17.10054717930957224, 11.04774946733758512 ) ) ;
#8445=CARTESIAN_POINT ( 'NONE',  ( 22.96512898726170704, 23.28924158689358848, 11.95042449705224819 ) ) ;
#8454=CARTESIAN_POINT ( 'NONE',  ( 3.903127820947815962E-15, 26.49999999999999289, 15.53125000000000355 ) ) ;
#8456=CARTESIAN_POINT ( 'NONE',  ( 22.47009348518006888, 19.30075366110858326, 13.00425721518280042 ) ) ;
#8458=CARTESIAN_POINT ( 'NONE',  ( 16.90694777372845437, 16.62861179130368683, 12.08020438729360180 ) ) ;
#8461=CARTESIAN_POINT ( 'NONE',  ( -2.500000000000004441, 28.96446609406725159, 15.29687500000000178 ) ) ;
#8472=CARTESIAN_POINT ( 'NONE',  ( 22.44007493706583745, 19.34731747087121434, 12.00579112326928133 ) ) ;
#8473=CARTESIAN_POINT ( 'NONE',  ( -1.035533905932742860, 32.50000000000000000, 14.98437500000000533 ) ) ;
#8502=CARTESIAN_POINT ( 'NONE',  ( 21.27550008773165047, 17.38841780631423362, 10.95195840513859231 ) ) ;
#8511=CARTESIAN_POINT ( 'NONE',  ( -1.383578242660655100, 26.47259180932604039, 14.45531658473306535 ) ) ;
#8515=CARTESIAN_POINT ( 'NONE',  ( 20.55933174294505861, 16.75535677129292722, 12.94889058896590583 ) ) ;
#8519=CARTESIAN_POINT ( 'NONE',  ( 18.62184541094303114, 16.98042197548449295, 12.02177981800743112 ) ) ;
#8521=CARTESIAN_POINT ( 'NONE',  ( 1.767766952966377314, 28.23223304703363112, 14.43750000000000178 ) ) ;
#8522=CARTESIAN_POINT ( 'NONE',  ( 16.58601566935799454, 18.36373179894816943, 12.17661548709639696 ) ) ;
#8532=CARTESIAN_POINT ( 'NONE',  ( 4.553649124439118623E-15, 27.49999999999999289, 15.53125000000000355 ) ) ;
#8545=CARTESIAN_POINT ( 'NONE',  ( 16.23246227876473213, 18.01017840835489991, 12.17661548709639696 ) ) ;
#8556=CARTESIAN_POINT ( 'NONE',  ( 21.30711663910541276, 17.34296610691914253, 11.95042449705224819 ) ) ;
#8563=CARTESIAN_POINT ( 'NONE',  ( 2.521662442312487151, 27.57191497400665270, 13.43969158473306713 ) ) ;
#8566=CARTESIAN_POINT ( 'NONE',  ( 19.90085419568980640, 16.36478119802090703, 11.95042571680015442 ) ) ;
#8568=CARTESIAN_POINT ( 'NONE',  ( 18.64799062861727563, 15.97503555906617123, 11.97707131907271005 ) ) ;
#8569=CARTESIAN_POINT ( 'NONE',  ( 16.35082997044643704, 18.59891749786092063, 12.19867189564230969 ) ) ;
#8572=CARTESIAN_POINT ( 'NONE',  ( -1.035533905932736420, 27.49999999999998934, 14.20312500000000355 ) ) ;
#8577=CARTESIAN_POINT ( 'NONE',  ( 17.86810043078960319, 17.16701444005803268, 12.06109941161078325 ) ) ;
#8579=CARTESIAN_POINT ( 'NONE',  ( 21.41951502703731691, 22.64547864373410135, 12.00579112326941988 ) ) ;
#8590=CARTESIAN_POINT ( 'NONE',  ( -1.720978244806810498, 31.81455566112594013, 16.06030841526693820 ) ) ;
#8614=CARTESIAN_POINT ( 'NONE',  ( 16.98270770525814299, 16.57081904430127395, 11.07189675232624104 ) ) ;
#8623=CARTESIAN_POINT ( 'NONE',  ( 2.428085025993350410, 32.52166244231248271, 13.75219158473306535 ) ) ;
#8626=CARTESIAN_POINT ( 'NONE',  ( 22.99351140629659795, 23.33806509665494389, 12.94889058896590583 ) ) ;
#8628=CARTESIAN_POINT ( 'NONE',  ( 17.20991452582289583, 17.73983294248524700, 12.11810441208646338 ) ) ;
#8631=CARTESIAN_POINT ( 'NONE',  ( 1.767766952966372429, 31.76776695296637598, 14.75000000000000355 ) ) ;
#8640=CARTESIAN_POINT ( 'NONE',  ( 1.035533905932737975, 32.50000000000000711, 14.82812500000000355 ) ) ;
#8648=CARTESIAN_POINT ( 'NONE',  ( -2.500000000000007550, 31.03553390593274486, 15.14062500000000355 ) ) ;
#8651=PLANE ( 'NONE',  #9551 ) ;
#8673=CARTESIAN_POINT ( 'NONE',  ( 23.54706165660595829, 18.96431965174070555, 11.95042449705224819 ) ) ;
#8682=CARTESIAN_POINT ( 'NONE',  ( 3.527408190673962274, 28.61642175733934934, 13.51781658473306713 ) ) ;
#8684=CARTESIAN_POINT ( 'NONE',  ( 20.15426471261298147, 16.54100339847095213, 11.95042283504686154 ) ) ;
#8686=CARTESIAN_POINT ( 'NONE',  ( 21.90605485701305000, 18.97586566459109392, 12.00579112326941988 ) ) ;
#8691=ORIENTED_EDGE ( 'NONE', *, *, #6748, .F. ) ;
#8704=CARTESIAN_POINT ( 'NONE',  ( -2.500000000000005773, 29.99999999999999645, 16.46875000000000355 ) ) ;
#8705=CARTESIAN_POINT ( 'NONE',  ( -1.767766952966370209, 28.23223304703362402, 15.37500000000000355 ) ) ;
#8720=CARTESIAN_POINT ( 'NONE',  ( 20.05583492806123758, 17.75628287944761396, 11.00732503135576401 ) ) ;
#8730=CARTESIAN_POINT ( 'NONE',  ( -2.527408190673963162, 30.96936468028755840, 12.89281658473306535 ) ) ;
#8732=CARTESIAN_POINT ( 'NONE',  ( 24.14247934234231963, 22.08663129433533001, 12.94889058896630019 ) ) ;
#8734=CARTESIAN_POINT ( 'NONE',  ( 21.25655365073496839, 18.52406763439849513, 12.00579112326941988 ) ) ;
#8749=CARTESIAN_POINT ( 'NONE',  ( 2.474873734152918558, 32.47487373415292211, 16.00000000000000355 ) ) ;
#8755=CARTESIAN_POINT ( 'NONE',  ( 1.767766952966372429, 31.76776695296637598, 14.75000000000000355 ) ) ;
#8756=DIRECTION ( 'NONE',  ( -0.9876851083892491667, -0.1564548710207423754, 0.000000000000000000 ) ) ;
#8773=CARTESIAN_POINT ( 'NONE',  ( 18.94282644159813955, 20.01493855567512625, 10.95195840513859231 ) ) ;
#8779=CARTESIAN_POINT ( 'NONE',  ( 0.06616922564517943584, 27.49999999999998934, 13.28344158473306713 ) ) ;
#8782=CARTESIAN_POINT ( 'NONE',  ( 22.86591953417209666, 18.42728137938113875, 11.95042449705224819 ) ) ;
#8786=CARTESIAN_POINT ( 'NONE',  ( 18.88912242859132107, 19.99746927611068870, 11.95042449705224819 ) ) ;
#8787=EDGE_CURVE ( 'NONE', #6331, #9431, #424, .T. ) ;
#8789=CARTESIAN_POINT ( 'NONE',  ( 16.70557116688603472, 16.82996273904517182, 13.10128505860060066 ) ) ;
#8791=SURFACE_STYLE_FILL_AREA ( #10466 ) ;
#8796=CARTESIAN_POINT ( 'NONE',  ( 15.88045857259785087, 19.06928889570832197, 12.24278471274156388 ) ) ;
#8810=CARTESIAN_POINT ( 'NONE',  ( 1.449747468305836673, 26.49999999999999289, 15.60937500000000711 ) ) ;
#8815=CARTESIAN_POINT ( 'NONE',  ( 1.101703131577913553, 32.47259180932605460, 15.82593341526694353 ) ) ;
#8817=CARTESIAN_POINT ( 'NONE',  ( 19.05040816462259556, 17.06282649731835122, 12.00984920396035172 ) ) ;
#8836=CARTESIAN_POINT ( 'NONE',  ( 17.82405332881840110, 17.21173750719964346, 11.06307126761931769 ) ) ;
#8842=( GEOMETRIC_REPRESENTATION_CONTEXT ( 3 ) GLOBAL_UNCERTAINTY_ASSIGNED_CONTEXT ( ( #198 ) ) GLOBAL_UNIT_ASSIGNED_CONTEXT ( ( #3270, #3217, #9995 ) ) REPRESENTATION_CONTEXT ( 'NONE', 'WORKASPACE' ) );
#8843=CARTESIAN_POINT ( 'NONE',  ( -1.720978244806803170, 28.18544433887405987, 13.12719158473306535 ) ) ;
#8847=CARTESIAN_POINT ( 'NONE',  ( 18.94282644159813955, 20.01493855567512625, 10.95195840513859231 ) ) ;
#8850=CARTESIAN_POINT ( 'NONE',  ( 17.83714238635922911, 17.16560587574106123, 13.06440897074317853 ) ) ;
#8861=CARTESIAN_POINT ( 'NONE',  ( 19.08509339279509831, 17.01892842213374735, 13.00828316275149099 ) ) ;
#8869=CARTESIAN_POINT ( 'NONE',  ( 2.474873734152918558, 32.47487373415292211, 13.50000000000000355 ) ) ;
#8874=CARTESIAN_POINT ( 'NONE',  ( 3.472591809326051937, 28.48408330604899419, 16.76343341526694175 ) ) ;
#8887=CARTESIAN_POINT ( 'NONE',  ( 19.48730207459019326, 19.05393922246431870, 11.95042449705224996 ) ) ;
#8888=CARTESIAN_POINT ( 'NONE',  ( 19.17195227357822773, 19.49818538049391492, 10.95195840513741636 ) ) ;
#8895=CARTESIAN_POINT ( 'NONE',  ( 2.500000000000006661, 30.06616922564517580, 14.84594158473306713 ) ) ;
#8897=CARTESIAN_POINT ( 'NONE',  ( 21.79510105275299026, 17.74985623046760708, 10.95195840513859231 ) ) ;
#8899=CARTESIAN_POINT ( 'NONE',  ( 20.39832466968983837, 22.29813831026750393, 13.00425721518307753 ) ) ;
#8906=CARTESIAN_POINT ( 'NONE',  ( 23.31827848602400621, 20.57738196266585362, 12.00579112326941988 ) ) ;
#8914=EDGE_CURVE ( 'NONE', #10270, #6331, #1238, .T. ) ;
#8915=CARTESIAN_POINT ( 'NONE',  ( -3.527408190673961386, 28.61642175733934224, 16.29468341526694530 ) ) ;
#8918=CARTESIAN_POINT ( 'NONE',  ( -2.527408190673963162, 29.03063531971243094, 15.04468341526694175 ) ) ;
#8936=CARTESIAN_POINT ( 'NONE',  ( 17.16312581766332457, 17.78662165064481471, 11.12029599681952519 ) ) ;
#8937=VERTEX_POINT ( 'NONE', #5858 ) ;
#8944=CARTESIAN_POINT ( 'NONE',  ( -1.767766952966375094, 31.76776695296636888, 15.06250000000000355 ) ) ;
#8946=CARTESIAN_POINT ( 'NONE',  ( 16.30404126228686579, 18.64570620602049189, 11.20086348037537327 ) ) ;
#8951=CARTESIAN_POINT ( 'NONE',  ( 22.48167088160742821, 22.45759571798082987, 13.00425721518307753 ) ) ;
#8960=CARTESIAN_POINT ( 'NONE',  ( 20.08745147943499987, 17.71083118005251933, 12.00579112326941988 ) ) ;
#8968=CARTESIAN_POINT ( 'NONE',  ( 1.515916693951011140, 26.52740819067395250, 13.36156658473306535 ) ) ;
#8970=UNCERTAINTY_MEASURE_WITH_UNIT (LENGTH_MEASURE( 1.000000000000000082E-05 ), #9737, 'distance_accuracy_value', 'NONE');
#8974=CARTESIAN_POINT ( 'NONE',  ( -2.472591809326051937, 31.10170313157791000, 17.38843341526693820 ) ) ;
#8986=PRODUCT_DEFINITION ( 'UNKNOWN', '', #5630, #2457 ) ;
#8994=CARTESIAN_POINT ( 'NONE',  ( 16.74199038346592872, 18.20775708483950694, 12.16198771834549497 ) ) ;
#9006=CARTESIAN_POINT ( 'NONE',  ( 19.32754978430113368, 16.15626933694376888, 10.95875375162450638 ) ) ;
#9010=CARTESIAN_POINT ( 'NONE',  ( 20.50876875457641546, 17.93645829877244680, 13.00425721518307576 ) ) ;
#9018=CARTESIAN_POINT ( 'NONE',  ( 18.65992412991285221, 16.93717640447601269, 13.02011930655217675 ) ) ;
#9024=CARTESIAN_POINT ( 'NONE',  ( -1.720978244806803170, 28.18544433887405987, 13.12719158473306535 ) ) ;
#9029=CARTESIAN_POINT ( 'NONE',  ( 2.472591809326055046, 28.89829686842209355, 15.51343341526694353 ) ) ;
#9038=CARTESIAN_POINT ( 'NONE',  ( 1.449747468305832898, 33.50000000000000000, 14.82812500000000355 ) ) ;
#9042=CARTESIAN_POINT ( 'NONE',  ( 20.73695268571362504, 18.16262921024512167, 12.00579112326941988 ) ) ;
#9051=CARTESIAN_POINT ( 'NONE',  ( 23.19605965318632457, 18.72439211931539660, 10.95195840513869179 ) ) ;
#9055=CARTESIAN_POINT ( 'NONE',  ( 17.78598590678423719, 16.10215687441832699, 12.01726674494117653 ) ) ;
#9060=CARTESIAN_POINT ( 'NONE',  ( -3.527408190673961386, 28.61642175733934224, 15.04468341526694175 ) ) ;
#9062=CARTESIAN_POINT ( 'NONE',  ( 20.50876875457641546, 17.93645829877244680, 13.00425721518307576 ) ) ;
#9068=CARTESIAN_POINT ( 'NONE',  ( -3.494791681227492397, 29.65833842083190675, 15.48578750830907147 ) ) ;
#9074=CARTESIAN_POINT ( 'NONE',  ( -2.472591809326051937, 31.10170313157791000, 14.88843341526694353 ) ) ;
#9084=CARTESIAN_POINT ( 'NONE',  ( -3.500000000000002665, 28.55025253169416288, 15.29687500000000533 ) ) ;
#9089=CARTESIAN_POINT ( 'NONE',  ( 17.59356678224322934, 17.35619608210146581, 12.08212522340233264 ) ) ;
#9095=DIRECTION ( 'NONE',  ( 0.6587175828649983744, -0.7523902883640206651, 4.024558464266192459E-16 ) ) ;
#9100=CARTESIAN_POINT ( 'NONE',  ( 16.35082997044643704, 18.59891749786092063, 12.19867189564230969 ) ) ;
#9104=CARTESIAN_POINT ( 'NONE',  ( 20.18549546789347460, 16.49528347911771675, 12.94888893485705061 ) ) ;
#9109=CARTESIAN_POINT ( 'NONE',  ( 1.449747468305836673, 26.49999999999999289, 14.35937500000000711 ) ) ;
#9112=CARTESIAN_POINT ( 'NONE',  ( 15.45532619834991017, 18.08020770756206019, 13.21853671947355302 ) ) ;
#9119=CARTESIAN_POINT ( 'NONE',  ( -3.500000000000001332, 29.93383077435482065, 15.47094158473306535 ) ) ;
#9128=CARTESIAN_POINT ( 'NONE',  ( 17.79249663040192431, 17.21067465782413919, 12.06642298039558980 ) ) ;
#9139=CARTESIAN_POINT ( 'NONE',  ( -2.474873734152916338, 27.52512626584707789, 15.37500000000000355 ) ) ;
#9145=CARTESIAN_POINT ( 'NONE',  ( 17.13192716875488131, 17.81782029955189728, 12.12541829646253078 ) ) ;
#9159=CARTESIAN_POINT ( 'NONE',  ( 19.32262643072814967, 17.24627075153934541, 11.00732576902737492 ) ) ;
#9161=CARTESIAN_POINT ( 'NONE',  ( 23.38258886820915095, 18.73219245557438484, 12.94889058896590583 ) ) ;
#9168=CARTESIAN_POINT ( 'NONE',  ( 17.31910053175343478, 17.63064693655086757, 11.10566822806672427 ) ) ;
#9169=CARTESIAN_POINT ( 'NONE',  ( 2.521662442312485819, 32.42808502599335441, 15.74780841526694175 ) ) ;
#9171=CARTESIAN_POINT ( 'NONE',  ( 19.93275388331568365, 16.31952634560019888, 12.94889180291853492 ) ) ;
#9177=CARTESIAN_POINT ( 'NONE',  ( -0.06616922564517727090, 32.50000000000000711, 12.65844158473306535 ) ) ;
#9184=COLOUR_RGB ( '', 0.40784314, 0.44705882, 0.49803922) ;
#9199=CARTESIAN_POINT ( 'NONE',  ( 4.553649124439118623E-15, 27.49999999999999289, 14.28125000000000355 ) ) ;
#9203=CARTESIAN_POINT ( 'NONE',  ( 16.89796509758404852, 18.05178237072099989, 12.14735994959144350 ) ) ;
#9212=CARTESIAN_POINT ( 'NONE',  ( -2.500000000000005773, 29.99999999999999645, 16.46875000000000355 ) ) ;
#9215=CARTESIAN_POINT ( 'NONE',  ( 17.40659673382103989, 17.54313596447427770, 11.09746175923963918 ) ) ;
#9219=CARTESIAN_POINT ( 'NONE',  ( 16.65878245872646701, 16.87675144720473952, 12.10347664333366247 ) ) ;
#9226=CARTESIAN_POINT ( 'NONE',  ( -3.500000000000003109, 29.99999999999999645, 13.96875000000000355 ) ) ;
#9228=CARTESIAN_POINT ( 'NONE',  ( 19.79543838746868190, 16.23930471839911149, 12.94973781945951785 ) ) ;
#9229=CARTESIAN_POINT ( 'NONE',  ( 22.08651808663882932, 17.88512374315008557, 11.95042449705224819 ) ) ;
#9232=CARTESIAN_POINT ( 'NONE',  ( 1.035533905932743970, 27.49999999999999289, 14.35937500000000711 ) ) ;
#9243=CARTESIAN_POINT ( 'NONE',  ( -1.767766952966370209, 28.23223304703362402, 15.37500000000000355 ) ) ;
#9257=DIRECTION ( 'NONE',  ( -0.7071067811865405783, -0.7071067811865545671, 0.000000000000000000 ) ) ;
#9269=CARTESIAN_POINT ( 'NONE',  ( 21.22493709936120254, 18.56951933379358621, 11.00732503135576401 ) ) ;
#9274=CARTESIAN_POINT ( 'NONE',  ( 18.81331750051067075, 21.67874213615617762, 12.94889058896551326 ) ) ;
#9281=CARTESIAN_POINT ( 'NONE',  ( 0.06616922564517879746, 26.50000000000000000, 14.53344158473306535 ) ) ;
#9283=CARTESIAN_POINT ( 'NONE',  ( 22.63773560303409127, 18.20111046790825782, 12.94889058896590583 ) ) ;
#9288=CARTESIAN_POINT ( 'NONE',  ( -1.035533905932736420, 27.49999999999998934, 15.45312500000000178 ) ) ;
#9296=CARTESIAN_POINT ( 'NONE',  ( 22.98009469009668138, 21.94211999725310491, 12.00579112326941988 ) ) ;
#9297=CARTESIAN_POINT ( 'NONE',  ( 1.035533905932743970, 27.49999999999999289, 14.35937500000000533 ) ) ;
#9327=CARTESIAN_POINT ( 'NONE',  ( 20.47715220320264962, 17.98190999816754498, 12.00579112326941988 ) ) ;
#9332=CARTESIAN_POINT ( 'NONE',  ( 16.14406960823794179, 17.39146429769401081, 11.14955153432450530 ) ) ;
#9342=CARTESIAN_POINT ( 'NONE',  ( -3.494791681227492397, 29.65833842083190675, 15.48578750830907147 ) ) ;
#9344=CARTESIAN_POINT ( 'NONE',  ( 22.48167088160742821, 22.45759571798082987, 13.00425721518307753 ) ) ;
#9347=CARTESIAN_POINT ( 'NONE',  ( 19.69775075566884226, 17.43975236193677603, 12.00579112326941988 ) ) ;
#9349=CARTESIAN_POINT ( 'NONE',  ( -1.035533905932742638, 32.50000000000000000, 16.23437500000000355 ) ) ;
#9361=CARTESIAN_POINT ( 'NONE',  ( 20.08745147943499987, 17.71083118005251933, 12.00579112326941988 ) ) ;
#9362=CARTESIAN_POINT ( 'NONE',  ( 2.500000000000010214, 28.96446609406726580, 15.76562500000000178 ) ) ;
#9388=CARTESIAN_POINT ( 'NONE',  ( 21.04731615659443733, 17.16224689484156585, 11.95042449705224819 ) ) ;
#9395=CARTESIAN_POINT ( 'NONE',  ( -3.500000000000001332, 29.93383077435482065, 12.97094158473306358 ) ) ;
#9397=CARTESIAN_POINT ( 'NONE',  ( 20.75790788474667181, 23.61206934513595357, 12.94889058896590583 ) ) ;
#9400=CARTESIAN_POINT ( 'NONE',  ( 17.39179625728592882, 16.28601130006924791, 12.04260150961189524 ) ) ;
#9401=CARTESIAN_POINT ( 'NONE',  ( 20.00651627240589647, 19.97666299463432438, 12.00579112326824216 ) ) ;
#9403=CARTESIAN_POINT ( 'NONE',  ( 2.500000000000006661, 30.06616922564517580, 14.84594158473306713 ) ) ;
#9407=ORIENTED_EDGE ( 'NONE', *, *, #10554, .T. ) ;
#9412=CARTESIAN_POINT ( 'NONE',  ( -2.500000000000007550, 31.03553390593274131, 15.14062500000000355 ) ) ;
#9431=VERTEX_POINT ( 'NONE', #8887 ) ;
#9440=CARTESIAN_POINT ( 'NONE',  ( 19.12295744889739879, 19.47009535162641569, 11.95042449705107224 ) ) ;
#9449=CARTESIAN_POINT ( 'NONE',  ( -3.500000000000003109, 29.99999999999999645, 15.21875000000000355 ) ) ;
#9453=CARTESIAN_POINT ( 'NONE',  ( 19.38445574543743177, 22.63941596627307362, 11.95042449705263898 ) ) ;
#9455=CARTESIAN_POINT ( 'NONE',  ( 20.73695268571362504, 18.16262921024512167, 12.00579112326941988 ) ) ;
#9476=CARTESIAN_POINT ( 'NONE',  ( -2.500000000000007550, 30.06616922564517580, 16.21655841526694175 ) ) ;
#9489=SHAPE_DEFINITION_REPRESENTATION ( #5201, #716 ) ;
#9497=CARTESIAN_POINT ( 'NONE',  ( 19.48730207459018970, 19.05393922246432226, 11.95042449705224996 ) ) ;
#9504=DIRECTION ( 'NONE',  ( -0.7071067811865479058, -0.7071067811865470176, 0.000000000000000000 ) ) ;
#9506=CARTESIAN_POINT ( 'NONE',  ( -3.527408190673960053, 31.38357824266065066, 15.39281658473306358 ) ) ;
#9509=CARTESIAN_POINT ( 'NONE',  ( 23.22881793621964874, 18.67973499377871960, 11.95042449705234588 ) ) ;
#9511=CARTESIAN_POINT ( 'NONE',  ( 23.17052989764754756, 21.62756661655841839, 12.00579112326981246 ) ) ;
#9533=CARTESIAN_POINT ( 'NONE',  ( -0.06616922564517033201, 27.49999999999998934, 16.52905841526693820 ) ) ;
#9534=FACE_OUTER_BOUND ( 'NONE', #3413, .T. ) ;
#9551=AXIS2_PLACEMENT_3D ( 'NONE', #1137, #5489, #8756 ) ;
#9555=CARTESIAN_POINT ( 'NONE',  ( 19.52039169078502212, 17.38380627596665562, 11.00732402621840578 ) ) ;
#9562=CARTESIAN_POINT ( 'NONE',  ( 1.814555661125942132, 28.27902175519319883, 13.43969158473306713 ) ) ;
#9564=CARTESIAN_POINT ( 'NONE',  ( 24.35722724902042202, 20.98982846826517346, 11.95042449705185739 ) ) ;
#9565=DIRECTION ( 'NONE',  ( 1.000000000000000000, 0.000000000000000000, 0.000000000000000000 ) ) ;
#9568=CARTESIAN_POINT ( 'NONE',  ( 18.10462311893278553, 17.05669763433401087, 12.04589798090090902 ) ) ;
#9570=( NAMED_UNIT ( * ) SI_UNIT ( $, .STERADIAN. ) SOLID_ANGLE_UNIT ( ) );
#9574=CARTESIAN_POINT ( 'NONE',  ( 17.13192716875488131, 17.81782029955189728, 12.12541829646253078 ) ) ;
#9576=( BOUNDED_SURFACE ( )  B_SPLINE_SURFACE ( 3, 3, ( 
 ( #8796, #4479, #7863, #235, #7028, #9574, #1182, #5358, #1124, #7919, #3533, #5197, #8577, #960, #2698, #4365, #6916, #10305, #6075, #10634, #3026, #613, #10680, #5577, #8960, #554, #8129, #7338, #451, #508, #1353, #9848, #7286, #6446, #7396, #3953, #10579, #3853, #6349, #8906, #4637, #394, #9743, #3124, #2240, #5632, #4009, #5524, #3796, #8177, #8022, #6289, #1297, #10727 ),
 ( #1243, #2135, #9905, #6502, #2917, #4691, #8070, #7236, #4751, #5470, #3904, #6400, #3073, #9686, #9794, #9018, #2183, #8861, #1409, #4801, #2079, #7181, #2295, #4851, #5686, #9062, #1457, #8224, #2975, #6559, #7453, #2341, #8456, #10007, #2462, #4912, #10842, #6785, #1567, #3233, #10180, #8395, #8284, #9344, #7567, #2397, #9958, #4242, #773, #2571, #4179, #4120, #671, #1739 ),
 ( #2511, #9112, #5135, #10070, #1509, #5078, #1, #10895, #5845, #6606, #5021, #10956, #5956, #3349, #5786, #4968, #4070, #6731, #837, #9228, #9171, #5900, #10790, #8515, #7509, #3289, #6671, #893, #10124, #1623, #9283, #7628, #1676, #3402, #8340, #4295, #3176, #5733, #719, #223, #1169, #8732, #4352, #8626, #118, #2686, #9397, #5186, #5346, #6175, #59, #6907, #4416, #9614 ),
 ( #3463, #2012, #7071, #6844, #10400, #6012, #6226, #6955, #1795, #1964, #7904, #7801, #10344, #3518, #1908, #5296, #2855, #4468, #10292, #1845, #8566, #8684, #1113, #2739, #7741, #2798, #7684, #5398, #175, #3571, #6113, #8782, #7850, #9509, #1058, #4516, #3620, #283, #5239, #7011, #9564, #3677, #10461, #10237, #2636, #948, #6062, #1004, #9453, #10566, #6275, #2067, #2227, #3062 ),
 ( #1286, #6492, #5514, #4739, #6392, #497, #384, #4790, #3893, #7277, #5674, #7168, #5456, #9835, #9670, #7958, #2963, #9006, #3942, #8167, #2906, #8012, #544, #7328, #2286, #6335, #3787, #8897, #7224, #7118, #10622, #4681, #2173, #9051, #9730, #8116, #2128, #10514, #8057, #10671, #335, #4572, #3015, #9894, #5622, #437, #10717, #9783, #1399, #3730, #1231, #8847, #3115, #3840 ),
 ( #4628, #5566, #8946, #1339, #6438, #10057, #9945, #9168, #9215, #4058, #597, #5885, #2444, #8439, #5833, #5773, #2329, #7439, #6769, #1608, #9159, #4896, #818, #2498, #4223, #10112, #4839, #9269, #3389, #3995, #1663, #5060, #1553, #2553, #7613, #5005, #6719, #8381, #8273, #10167, #6593, #3165, #8215, #9994, #3269, #5938, #1446, #6653, #657, #7386, #10775, #6549, #5722, #8328 ),
 ( #10831, #3216, #9100, #1494, #2380, #4957, #706, #4108, #7494, #10880, #757, #4158, #7553, #10940, #3331, #7933, #3502, #8817, #8036, #310, #2991, #6888, #2933, #6310, #1781, #9327, #10220, #1720, #2037, #5225, #7200, #6250, #4335, #4280, #2617, #9643, #10595, #2877, #7986, #7724, #5430, #3447, #3705, #1259, #7143, #44, #10276, #5119, #7669, #2673, #10485, #7094, #4546, #10538 ) ),
 .UNSPECIFIED., .T., .F., .F. ) 
 B_SPLINE_SURFACE_WITH_KNOTS ( ( 4, 3, 4 ),
 ( 4, 2, 2, 2, 2, 2, 2, 2, 2, 2, 2, 2, 2, 2, 2, 2, 2, 2, 2, 2, 2, 2, 2, 2, 2, 2, 4 ),
 ( 0.000000000000000000, 0.5000000000000000000, 1.000000000000000000 ),
 ( 0.000000000000000000, 0.05059550242166081097, 0.08415034466705637040, 0.1009277657897541536, 0.1177051869124519229, 0.1353321994541143436, 0.1529592119957767782, 0.1882132370791016474, 0.2234672621624265165, 0.2410942747040889511, 0.2587212872457513857, 0.2827395206004625905, 0.3067577539551737398, 0.3547942206645960939, 0.4028306873740183924, 0.4268489207287295972, 0.4508671540834407465, 0.4680275555183331937, 0.4851879569532256964, 0.5195087598230107018, 0.5881503655625806015, 0.6567919713021505013, 0.7254335770417204010, 0.7940751827812903008, 0.8627167885208602005, 0.9313583942604301003, 1.000000000000000000 ),
 .UNSPECIFIED. ) 
 GEOMETRIC_REPRESENTATION_ITEM ( )  RATIONAL_B_SPLINE_SURFACE ( (
 ( 1.000000000000000000, 1.000000000000000000, 1.000000000000000000, 1.000000000000000000, 1.000000000000000000, 1.000000000000000000, 1.000000000000000000, 1.000000000000000000, 1.000000000000000000, 1.000000000000000000, 1.000000000000000000, 1.000000000000000000, 1.000000000000000000, 1.000000000000000000, 1.000000000000000000, 1.000000000000000000, 1.000000000000000000, 1.000000000000000000, 1.000000000000000000, 1.000000000000000000, 1.000000000000000000, 1.000000000000000000, 1.000000000000000000, 1.000000000000000000, 1.000000000000000000, 1.000000000000000000, 1.000000000000000000, 1.000000000000000000, 1.000000000000000000, 1.000000000000000000, 1.000000000000000000, 1.000000000000000000, 1.000000000000000000, 1.000000000000000000, 1.000000000000000000, 1.000000000000000000, 1.000000000000000000, 1.000000000000000000, 1.000000000000000000, 1.000000000000000000, 1.000000000000000000, 1.000000000000000000, 1.000000000000000000, 1.000000000000000000, 1.000000000000000000, 1.000000000000000000, 1.000000000000000000, 1.000000000000000000, 1.000000000000000000, 1.000000000000000000, 1.000000000000000000, 1.000000000000000000, 1.000000000000000000, 1.000000000000000000),
 ( 0.3333333333333333703, 0.3333333333333333703, 0.3333333333333333703, 0.3333333333333333703, 0.3333333333333333703, 0.3333333333333333703, 0.3333333333333333703, 0.3333333333333333703, 0.3333333333333333703, 0.3333333333333333703, 0.3333333333333333703, 0.3333333333333333703, 0.3333333333333333703, 0.3333333333333333703, 0.3333333333333333703, 0.3333333333333333703, 0.3333333333333333703, 0.3333333333333333703, 0.3333333333333333703, 0.3333333333333333703, 0.3333333333333333703, 0.3333333333333333703, 0.3333333333333333703, 0.3333333333333333703, 0.3333333333333333703, 0.3333333333333333703, 0.3333333333333333703, 0.3333333333333333703, 0.3333333333333333703, 0.3333333333333333703, 0.3333333333333333703, 0.3333333333333333703, 0.3333333333333333703, 0.3333333333333333703, 0.3333333333333333703, 0.3333333333333333703, 0.3333333333333333703, 0.3333333333333333703, 0.3333333333333333703, 0.3333333333333333703, 0.3333333333333333703, 0.3333333333333333703, 0.3333333333333333703, 0.3333333333333333703, 0.3333333333333333703, 0.3333333333333333703, 0.3333333333333333703, 0.3333333333333333703, 0.3333333333333333703, 0.3333333333333333703, 0.3333333333333333703, 0.3333333333333333703, 0.3333333333333333703, 0.3333333333333333703),
 ( 0.3333333333333333703, 0.3333333333333333703, 0.3333333333333333703, 0.3333333333333333703, 0.3333333333333333703, 0.3333333333333333703, 0.3333333333333333703, 0.3333333333333333703, 0.3333333333333333703, 0.3333333333333333703, 0.3333333333333333703, 0.3333333333333333703, 0.3333333333333333703, 0.3333333333333333703, 0.3333333333333333703, 0.3333333333333333703, 0.3333333333333333703, 0.3333333333333333703, 0.3333333333333333703, 0.3333333333333333703, 0.3333333333333333703, 0.3333333333333333703, 0.3333333333333333703, 0.3333333333333333703, 0.3333333333333333703, 0.3333333333333333703, 0.3333333333333333703, 0.3333333333333333703, 0.3333333333333333703, 0.3333333333333333703, 0.3333333333333333703, 0.3333333333333333703, 0.3333333333333333703, 0.3333333333333333703, 0.3333333333333333703, 0.3333333333333333703, 0.3333333333333333703, 0.3333333333333333703, 0.3333333333333333703, 0.3333333333333333703, 0.3333333333333333703, 0.3333333333333333703, 0.3333333333333333703, 0.3333333333333333703, 0.3333333333333333703, 0.3333333333333333703, 0.3333333333333333703, 0.3333333333333333703, 0.3333333333333333703, 0.3333333333333333703, 0.3333333333333333703, 0.3333333333333333703, 0.3333333333333333703, 0.3333333333333333703),
 ( 1.000000000000000000, 1.000000000000000000, 1.000000000000000000, 1.000000000000000000, 1.000000000000000000, 1.000000000000000000, 1.000000000000000000, 1.000000000000000000, 1.000000000000000000, 1.000000000000000000, 1.000000000000000000, 1.000000000000000000, 1.000000000000000000, 1.000000000000000000, 1.000000000000000000, 1.000000000000000000, 1.000000000000000000, 1.000000000000000000, 1.000000000000000000, 1.000000000000000000, 1.000000000000000000, 1.000000000000000000, 1.000000000000000000, 1.000000000000000000, 1.000000000000000000, 1.000000000000000000, 1.000000000000000000, 1.000000000000000000, 1.000000000000000000, 1.000000000000000000, 1.000000000000000000, 1.000000000000000000, 1.000000000000000000, 1.000000000000000000, 1.000000000000000000, 1.000000000000000000, 1.000000000000000000, 1.000000000000000000, 1.000000000000000000, 1.000000000000000000, 1.000000000000000000, 1.000000000000000000, 1.000000000000000000, 1.000000000000000000, 1.000000000000000000, 1.000000000000000000, 1.000000000000000000, 1.000000000000000000, 1.000000000000000000, 1.000000000000000000, 1.000000000000000000, 1.000000000000000000, 1.000000000000000000, 1.000000000000000000),
 ( 0.3333333333333333703, 0.3333333333333333703, 0.3333333333333333703, 0.3333333333333333703, 0.3333333333333333703, 0.3333333333333333703, 0.3333333333333333703, 0.3333333333333333703, 0.3333333333333333703, 0.3333333333333333703, 0.3333333333333333703, 0.3333333333333333703, 0.3333333333333333703, 0.3333333333333333703, 0.3333333333333333703, 0.3333333333333333703, 0.3333333333333333703, 0.3333333333333333703, 0.3333333333333333703, 0.3333333333333333703, 0.3333333333333333703, 0.3333333333333333703, 0.3333333333333333703, 0.3333333333333333703, 0.3333333333333333703, 0.3333333333333333703, 0.3333333333333333703, 0.3333333333333333703, 0.3333333333333333703, 0.3333333333333333703, 0.3333333333333333703, 0.3333333333333333703, 0.3333333333333333703, 0.3333333333333333703, 0.3333333333333333703, 0.3333333333333333703, 0.3333333333333333703, 0.3333333333333333703, 0.3333333333333333703, 0.3333333333333333703, 0.3333333333333333703, 0.3333333333333333703, 0.3333333333333333703, 0.3333333333333333703, 0.3333333333333333703, 0.3333333333333333703, 0.3333333333333333703, 0.3333333333333333703, 0.3333333333333333703, 0.3333333333333333703, 0.3333333333333333703, 0.3333333333333333703, 0.3333333333333333703, 0.3333333333333333703),
 ( 0.3333333333333333703, 0.3333333333333333703, 0.3333333333333333703, 0.3333333333333333703, 0.3333333333333333703, 0.3333333333333333703, 0.3333333333333333703, 0.3333333333333333703, 0.3333333333333333703, 0.3333333333333333703, 0.3333333333333333703, 0.3333333333333333703, 0.3333333333333333703, 0.3333333333333333703, 0.3333333333333333703, 0.3333333333333333703, 0.3333333333333333703, 0.3333333333333333703, 0.3333333333333333703, 0.3333333333333333703, 0.3333333333333333703, 0.3333333333333333703, 0.3333333333333333703, 0.3333333333333333703, 0.3333333333333333703, 0.3333333333333333703, 0.3333333333333333703, 0.3333333333333333703, 0.3333333333333333703, 0.3333333333333333703, 0.3333333333333333703, 0.3333333333333333703, 0.3333333333333333703, 0.3333333333333333703, 0.3333333333333333703, 0.3333333333333333703, 0.3333333333333333703, 0.3333333333333333703, 0.3333333333333333703, 0.3333333333333333703, 0.3333333333333333703, 0.3333333333333333703, 0.3333333333333333703, 0.3333333333333333703, 0.3333333333333333703, 0.3333333333333333703, 0.3333333333333333703, 0.3333333333333333703, 0.3333333333333333703, 0.3333333333333333703, 0.3333333333333333703, 0.3333333333333333703, 0.3333333333333333703, 0.3333333333333333703),
 ( 1.000000000000000000, 1.000000000000000000, 1.000000000000000000, 1.000000000000000000, 1.000000000000000000, 1.000000000000000000, 1.000000000000000000, 1.000000000000000000, 1.000000000000000000, 1.000000000000000000, 1.000000000000000000, 1.000000000000000000, 1.000000000000000000, 1.000000000000000000, 1.000000000000000000, 1.000000000000000000, 1.000000000000000000, 1.000000000000000000, 1.000000000000000000, 1.000000000000000000, 1.000000000000000000, 1.000000000000000000, 1.000000000000000000, 1.000000000000000000, 1.000000000000000000, 1.000000000000000000, 1.000000000000000000, 1.000000000000000000, 1.000000000000000000, 1.000000000000000000, 1.000000000000000000, 1.000000000000000000, 1.000000000000000000, 1.000000000000000000, 1.000000000000000000, 1.000000000000000000, 1.000000000000000000, 1.000000000000000000, 1.000000000000000000, 1.000000000000000000, 1.000000000000000000, 1.000000000000000000, 1.000000000000000000, 1.000000000000000000, 1.000000000000000000, 1.000000000000000000, 1.000000000000000000, 1.000000000000000000, 1.000000000000000000, 1.000000000000000000, 1.000000000000000000, 1.000000000000000000, 1.000000000000000000, 1.000000000000000000) ) ) 
 REPRESENTATION_ITEM ( '' )  SURFACE ( )  );
#9580=CARTESIAN_POINT ( 'NONE',  ( 3.500000000000005773, 31.44974746830583356, 15.92187500000000178 ) ) ;
#9584=CARTESIAN_POINT ( 'NONE',  ( 2.500000000000007550, 31.03553390593274486, 14.67187500000000178 ) ) ;
#9602=CARTESIAN_POINT ( 'NONE',  ( 23.08245441082096150, 20.10811672198468969, 11.00732503135576401 ) ) ;
#9611=CARTESIAN_POINT ( 'NONE',  ( 0.9693646802875628410, 32.52740819067395961, 13.83031658473306535 ) ) ;
#9614=CARTESIAN_POINT ( 'NONE',  ( 19.44564476272491049, 19.01746825227115067, 12.94889058896590761 ) ) ;
#9619=CARTESIAN_POINT ( 'NONE',  ( 16.39761867860600475, 18.55212878970134938, 13.19648031090924789 ) ) ;
#9637=CARTESIAN_POINT ( 'NONE',  ( 1.515916693951008254, 33.47259180932604750, 17.07593341526694530 ) ) ;
#9640=CARTESIAN_POINT ( 'NONE',  ( -1.767766952966375094, 31.76776695296636888, 15.06250000000000355 ) ) ;
#9642=CARTESIAN_POINT ( 'NONE',  ( 1.035533905932737975, 32.50000000000000711, 14.82812500000000178 ) ) ;
#9643=CARTESIAN_POINT ( 'NONE',  ( 22.82387490247590733, 19.65457484615246386, 12.00579112326941988 ) ) ;
#9660=CARTESIAN_POINT ( 'NONE',  ( 22.42093126068789033, 23.47289781856171587, 10.95195840513859231 ) ) ;
#9668=CARTESIAN_POINT ( 'NONE',  ( 1.814555661125942132, 28.27902175519319883, 14.68969158473306535 ) ) ;
#9670=CARTESIAN_POINT ( 'NONE',  ( 18.02930464311577907, 16.06944570838860642, 11.00389976449426399 ) ) ;
#9677=CARTESIAN_POINT ( 'NONE',  ( 23.18216631463591781, 20.05868775325893338, 13.00425721518307753 ) ) ;
#9686=CARTESIAN_POINT ( 'NONE',  ( 18.14679736200770677, 17.01284808935846371, 13.04404649446423115 ) ) ;
#9695=CARTESIAN_POINT ( 'NONE',  ( -2.474873734152920335, 32.47487373415291501, 15.06250000000000355 ) ) ;
#9700=CARTESIAN_POINT ( 'NONE',  ( 3.500000000000007994, 29.93383077435482420, 16.84155841526694175 ) ) ;
#9701=CARTESIAN_POINT ( 'NONE',  ( 2.500000000000007550, 31.03553390593274486, 15.92187500000000178 ) ) ;
#9719=CARTESIAN_POINT ( 'NONE',  ( 23.50695973324029353, 19.00259546466308791, 10.95195840513859231 ) ) ;
#9726=CARTESIAN_POINT ( 'NONE',  ( 2.500000000000010214, 28.96446609406726225, 14.51562500000000355 ) ) ;
#9730=CARTESIAN_POINT ( 'NONE',  ( 23.31046218964701211, 18.81639786330068276, 10.95195840513859231 ) ) ;
#9735=CARTESIAN_POINT ( 'NONE',  ( 23.37401553338360571, 20.56828919810574519, 13.00425721518307753 ) ) ;
#9737=( LENGTH_UNIT ( ) NAMED_UNIT ( * ) SI_UNIT ( .MILLI., .METRE. ) );
#9743=CARTESIAN_POINT ( 'NONE',  ( 22.98009469009668138, 21.94211999725310491, 12.00579112326941988 ) ) ;
#9751=CARTESIAN_POINT ( 'NONE',  ( 3.500000000000007994, 28.55025253169416644, 14.51562500000000355 ) ) ;
#9756=CARTESIAN_POINT ( 'NONE',  ( 1.515916693951008254, 33.47259180932604750, 15.82593341526694353 ) ) ;
#9757=CARTESIAN_POINT ( 'NONE',  ( 1.814555661125939467, 31.72097824480680828, 16.99780841526693820 ) ) ;
#9773=CARTESIAN_POINT ( 'NONE',  ( 18.06244887585786074, 17.10054717930957224, 11.04774946733758512 ) ) ;
#9779=CARTESIAN_POINT ( 'NONE',  ( 1.767766952966377314, 28.23223304703363112, 14.43750000000000178 ) ) ;
#9783=CARTESIAN_POINT ( 'NONE',  ( 19.82941471729559524, 23.00258574805652856, 10.95195840513859231 ) ) ;
#9785=CARTESIAN_POINT ( 'NONE',  ( 15.45532619834991017, 18.08020770756206019, 13.21853671947355302 ) ) ;
#9794=CARTESIAN_POINT ( 'NONE',  ( 18.31593954903570776, 16.96748919427588831, 13.03503021400358541 ) ) ;
#9802=CARTESIAN_POINT ( 'NONE',  ( 2.428085025993350410, 32.52166244231248271, 12.50219158473306358 ) ) ;
#9807=CARTESIAN_POINT ( 'NONE',  ( -0.9693646802875689472, 32.52740819067395961, 15.98218341526694175 ) ) ;
#9810=CARTESIAN_POINT ( 'NONE',  ( 16.58601566935801586, 18.36373179894819074, 12.17661548709639696 ) ) ;
#9827=CARTESIAN_POINT ( 'NONE',  ( 23.31827848602400621, 20.57738196266585362, 12.00579112326941988 ) ) ;
#9835=CARTESIAN_POINT ( 'NONE',  ( 17.74381166370891449, 16.14600641939347980, 11.01911823137775492 ) ) ;
#9841=CARTESIAN_POINT ( 'NONE',  ( 17.69587633286529282, 17.26453111358909354, 13.07531547515800874 ) ) ;
#9848=CARTESIAN_POINT ( 'NONE',  ( 22.29575558078030895, 19.24694448270711788, 12.00579112326941988 ) ) ;
#9855=AXIS2_PLACEMENT_3D ( 'NONE', #4951, #9095, #4785 ) ;
#9857=CARTESIAN_POINT ( 'NONE',  ( 2.521662442312487151, 27.57191497400665270, 13.43969158473306713 ) ) ;
#9863=CARTESIAN_POINT ( 'NONE',  ( 1.101703131577913553, 32.47259180932605460, 15.82593341526694353 ) ) ;
#9881=CARTESIAN_POINT ( 'NONE',  ( 19.95755123817951215, 17.62047157401400810, 12.00579112326941988 ) ) ;
#9890=CARTESIAN_POINT ( 'NONE',  ( 2.500000000000008438, 30.00000000000000711, 15.84375000000000355 ) ) ;
#9894=CARTESIAN_POINT ( 'NONE',  ( 22.93674656822681612, 23.24041807713223307, 10.95195840513859231 ) ) ;
#9897=CARTESIAN_POINT ( 'NONE',  ( 17.26579466391090634, 16.35877559204224951, 12.05147379044805866 ) ) ;
#9905=CARTESIAN_POINT ( 'NONE',  ( 16.39761867860600475, 18.55212878970134938, 13.19648031090924789 ) ) ;
#9912=CARTESIAN_POINT ( 'NONE',  ( -2.469212770973128190, 29.60886282244813827, 16.49922112211940117 ) ) ;
#9913=CARTESIAN_POINT ( 'NONE',  ( -1.814555661125939912, 31.72097824480680117, 12.81469158473306713 ) ) ;
#9918=CARTESIAN_POINT ( 'NONE',  ( -1.101703131577911776, 27.52740819067395250, 15.20093341526694353 ) ) ;
#9927=CARTESIAN_POINT ( 'NONE',  ( 2.474873734152918558, 32.47487373415292211, 14.75000000000000355 ) ) ;
#9933=CARTESIAN_POINT ( 'NONE',  ( 19.83233192245754140, 21.00689442486442360, 11.00732503135576401 ) ) ;
#9945=CARTESIAN_POINT ( 'NONE',  ( 17.16312581766332457, 17.78662165064481471, 11.12029599681952519 ) ) ;
#9949=CARTESIAN_POINT ( 'NONE',  ( 18.07012887690021330, 16.02595819568259827, 12.00212024154935975 ) ) ;
#9950=EDGE_CURVE ( 'NONE', #7325, #2956, #7685, .T. ) ;
#9954=CARTESIAN_POINT ( 'NONE',  ( -2.474873734152920335, 32.47487373415291501, 13.81250000000000355 ) ) ;
#9958=CARTESIAN_POINT ( 'NONE',  ( 21.04196501824306864, 22.63405165899350635, 13.00425721518307753 ) ) ;
#9963=CARTESIAN_POINT ( 'NONE',  ( 0.06616922564517943584, 27.49999999999998934, 14.53344158473306535 ) ) ;
#9968=CARTESIAN_POINT ( 'NONE',  ( 1.383578242660662871, 26.47259180932604039, 15.35718341526694530 ) ) ;
#9978=CARTESIAN_POINT ( 'NONE',  ( 2.474873734152922111, 27.52512626584708144, 14.43750000000000178 ) ) ;
#9984=CARTESIAN_POINT ( 'NONE',  ( 20.21677217982034946, 21.95921345637081501, 11.00732503135595941 ) ) ;
#9994=CARTESIAN_POINT ( 'NONE',  ( 22.42490604353609029, 22.35994869845890065, 11.00732503135576401 ) ) ;
#9995=( NAMED_UNIT ( * ) SI_UNIT ( $, .STERADIAN. ) SOLID_ANGLE_UNIT ( ) );
#9999=CARTESIAN_POINT ( 'NONE',  ( 19.93275388331568365, 16.31952634560019888, 12.94889180291853492 ) ) ;
#10005=CARTESIAN_POINT ( 'NONE',  ( -2.521662442312483599, 27.57191497400664204, 16.37280841526694175 ) ) ;
#10007=CARTESIAN_POINT ( 'NONE',  ( 22.67082259973814828, 19.44041185113230341, 13.00425721518326938 ) ) ;
#10015=CARTESIAN_POINT ( 'NONE',  ( -2.428085025993349078, 27.47833755768751374, 14.37719158473306713 ) ) ;
#10026=CARTESIAN_POINT ( 'NONE',  ( 17.86810043078960319, 17.16701444005803268, 12.06109941161078325 ) ) ;
#10036=CARTESIAN_POINT ( 'NONE',  ( -3.500000000000003997, 31.44974746830583001, 13.89062500000000355 ) ) ;
#10044=CARTESIAN_POINT ( 'NONE',  ( 20.17304365239387565, 21.99495017005343200, 12.00579112326981068 ) ) ;
#10057=CARTESIAN_POINT ( 'NONE',  ( 17.08513846059531005, 17.86460900771146143, 11.12760988119559258 ) ) ;
#10058=SURFACE_SIDE_STYLE ('',( #2446 ) ) ;
#10060=CARTESIAN_POINT ( 'NONE',  ( 16.19085831639751305, 17.34467558953444311, 12.14735994959144350 ) ) ;
#10067=CARTESIAN_POINT ( 'NONE',  ( -2.505208318772514708, 29.86938897312880314, 17.48140433884295319 ) ) ;
#10070=CARTESIAN_POINT ( 'NONE',  ( 16.08167231043895384, 17.45386159549338245, 13.15979613361243494 ) ) ;
#10071=CARTESIAN_POINT ( 'NONE',  ( 21.04731615659443733, 17.16224689484156585, 11.95042449705224819 ) ) ;
#10072=CIRCLE ( 'NONE', #6698, 0.4999999999999985567 ) ;
#10073=CIRCLE ( 'NONE', #484, 0.4999999999999981681 ) ;
#10076=CARTESIAN_POINT ( 'NONE',  ( 2.428085025993350410, 32.52166244231248271, 13.75219158473306535 ) ) ;
#10088=CARTESIAN_POINT ( 'NONE',  ( 2.500000000000010214, 28.96446609406726580, 14.51562500000000355 ) ) ;
#10112=CARTESIAN_POINT ( 'NONE',  ( 20.44553565182888732, 18.02736169756263962, 11.00732503135576401 ) ) ;
#10115=CARTESIAN_POINT ( 'NONE',  ( 23.94195266346560658, 19.36439822498074648, 12.94889058896590583 ) ) ;
#10122=CARTESIAN_POINT ( 'NONE',  ( -3.500000000000003553, 31.44974746830583356, 15.14062500000000355 ) ) ;
#10124=CARTESIAN_POINT ( 'NONE',  ( 22.11813463801259161, 17.83967204375498383, 12.94889058896590583 ) ) ;
#10129=CARTESIAN_POINT ( 'NONE',  ( -1.035533905932742638, 32.50000000000000000, 14.98437500000000711 ) ) ;
#10139=CARTESIAN_POINT ( 'NONE',  ( 20.23853826540680600, 19.71164639310234534, 12.00579112326941988 ) ) ;
#10156=FACE_OUTER_BOUND ( 'NONE', #3795, .T. ) ;
#10167=CARTESIAN_POINT ( 'NONE',  ( 23.26254143866440671, 20.58647472722595850, 11.00732503135576401 ) ) ;
#10172=CARTESIAN_POINT ( 'NONE',  ( 15.12656308325174415, 18.40897082268132934, 11.24497629747462568 ) ) ;
#10177=ORIENTED_EDGE ( 'NONE', *, *, #10452, .F. ) ;
#10178=CARTESIAN_POINT ( 'NONE',  ( -3.500000000000001332, 29.93383077435482065, 15.47094158473306535 ) ) ;
#10180=CARTESIAN_POINT ( 'NONE',  ( 23.39622245855813176, 20.94697541805627239, 13.00425721518248956 ) ) ;
#10182=CARTESIAN_POINT ( 'NONE',  ( 22.11805565807571128, 22.55986279155152374, 12.00579112326941988 ) ) ;
#10184=CARTESIAN_POINT ( 'NONE',  ( 1.767766952966377314, 28.23223304703363112, 15.68750000000000355 ) ) ;
#10193=CARTESIAN_POINT ( 'NONE',  ( 21.90605485701305000, 18.97586566459109392, 12.00579112326941988 ) ) ;
#10194=CARTESIAN_POINT ( 'NONE',  ( 1.767766952966377314, 28.23223304703363112, 15.68750000000000355 ) ) ;
#10217=PRODUCT_CONTEXT ( 'NONE', #1170, 'mechanical' ) ;
#10220=CARTESIAN_POINT ( 'NONE',  ( 20.73695268571362504, 18.16262921024512167, 12.00579112326941988 ) ) ;
#10226=CARTESIAN_POINT ( 'NONE',  ( 21.34179237787287065, 23.66094220255952152, 11.95042449705224819 ) ) ;
#10235=CARTESIAN_POINT ( 'NONE',  ( -3.500000000000003109, 29.99999999999999645, 16.46875000000000355 ) ) ;
#10237=CARTESIAN_POINT ( 'NONE',  ( 22.96512898726170704, 23.28924158689358848, 11.95042449705224819 ) ) ;
#10240=CARTESIAN_POINT ( 'NONE',  ( 17.26579466391090634, 16.35877559204224951, 12.05147379044805866 ) ) ;
#10241=CARTESIAN_POINT ( 'NONE',  ( 18.27511531525127353, 17.01097670698189290, 12.03680973694848966 ) ) ;
#10243=CARTESIAN_POINT ( 'NONE',  ( -2.500000000000005773, 29.99999999999999645, 16.46875000000000355 ) ) ;
#10253=CARTESIAN_POINT ( 'NONE',  ( 21.25655365073496839, 18.52406763439849513, 12.00579112326941988 ) ) ;
#10254=CARTESIAN_POINT ( 'NONE',  ( 1.035533905932743970, 27.49999999999999289, 15.60937500000000533 ) ) ;
#10261=CARTESIAN_POINT ( 'NONE',  ( -2.385244779468109755E-15, 32.50000000000000711, 13.65625000000000355 ) ) ;
#10265=STYLED_ITEM ( 'NONE', ( #3792 ), #5271 ) ;
#10270=VERTEX_POINT ( 'NONE', #5687 ) ;
#10276=CARTESIAN_POINT ( 'NONE',  ( 21.05771646464872404, 22.57981893131178452, 12.00579112326941988 ) ) ;
#10281=CARTESIAN_POINT ( 'NONE',  ( 24.32342464814431438, 20.41340561598360992, 11.95042449705224996 ) ) ;
#10290=CARTESIAN_POINT ( 'NONE',  ( -1.734723475976807094E-15, 33.50000000000000000, 14.90625000000000355 ) ) ;
#10292=CARTESIAN_POINT ( 'NONE',  ( 19.49929303312607942, 16.16195407633872350, 11.95465698723049108 ) ) ;
#10295=CARTESIAN_POINT ( 'NONE',  ( 19.49929303312607942, 16.16195407633872350, 11.95465698723049108 ) ) ;
#10296=CARTESIAN_POINT ( 'NONE',  ( 22.88317621546045189, 19.71992003298075957, 12.00579112326941988 ) ) ;
#10298=CARTESIAN_POINT ( 'NONE',  ( -2.500000000000007550, 31.03553390593274486, 16.39062500000000355 ) ) ;
#10305=CARTESIAN_POINT ( 'NONE',  ( 19.05040816462259556, 17.06282649731835122, 12.00984920396035172 ) ) ;
#10307=CARTESIAN_POINT ( 'NONE',  ( 19.69775075566884226, 17.43975236193677603, 12.00579112326941988 ) ) ;
#10308=CARTESIAN_POINT ( 'NONE',  ( 1.767766952966377314, 28.23223304703363112, 14.43750000000000178 ) ) ;
#10311=DIRECTION ( 'NONE',  ( 0.6587175828649982634, -0.7523902883640206651, 3.989863994746656317E-16 ) ) ;
#10317=CARTESIAN_POINT ( 'NONE',  ( 4.553649124439118623E-15, 27.49999999999999289, 15.53125000000000355 ) ) ;
#10318=CARTESIAN_POINT ( 'NONE',  ( -2.500000000000007550, 31.03553390593274486, 15.14062500000000355 ) ) ;
#10324=DIRECTION ( 'NONE',  ( -0.7055570967602625698, 0.7055570967602456944, 0.06616922564518108729 ) ) ;
#10334=CARTESIAN_POINT ( 'NONE',  ( 22.98142095123195716, 18.50759888342988546, 11.95042449705211141 ) ) ;
#10340=PRODUCT ( 'Tension Return Spring', 'Tension Return Spring', '', ( #10217 ) ) ;
#10342=CARTESIAN_POINT ( 'NONE',  ( -3.500000000000002665, 29.72450764647708255, 16.48359592357600434 ) ) ;
#10343=ORIENTED_EDGE ( 'NONE', *, *, #8787, .F. ) ;
#10344=CARTESIAN_POINT ( 'NONE',  ( 17.39179625728592882, 16.28601130006924791, 12.04260150961189524 ) ) ;
#10347=CARTESIAN_POINT ( 'NONE',  ( 22.98009469009668138, 21.94211999725310491, 12.00579112326941988 ) ) ;
#10349=CARTESIAN_POINT ( 'NONE',  ( -1.035533905932742638, 32.50000000000000000, 13.73437500000000533 ) ) ;
#10368=CARTESIAN_POINT ( 'NONE',  ( 2.500000000000008438, 30.00000000000000711, 15.84375000000000355 ) ) ;
#10369=CARTESIAN_POINT ( 'NONE',  ( -2.385244779468109755E-15, 32.50000000000000711, 16.15625000000000355 ) ) ;
#10373=LINE ( 'NONE', #4389, #1625 ) ;
#10389=CARTESIAN_POINT ( 'NONE',  ( 24.03139851132786831, 19.63770821034670533, 11.95042449705224996 ) ) ;
#10397=CARTESIAN_POINT ( 'NONE',  ( 0.9693646802875628410, 32.52740819067395961, 12.58031658473306713 ) ) ;
#10400=CARTESIAN_POINT ( 'NONE',  ( 16.19085831639751305, 17.34467558953444311, 12.14735994959144350 ) ) ;
#10402=CARTESIAN_POINT ( 'NONE',  ( 20.47715220320264962, 17.98190999816754498, 12.00579112326941988 ) ) ;
#10423=CARTESIAN_POINT ( 'NONE',  ( 1.449747468305833120, 33.50000000000000000, 14.82812500000000178 ) ) ;
#10427=CARTESIAN_POINT ( 'NONE',  ( -1.720978244806810498, 31.81455566112594013, 14.81030841526694175 ) ) ;
#10431=CARTESIAN_POINT ( 'NONE',  ( -2.469212770973128190, 29.60886282244813117, 16.49922112211940117 ) ) ;
#10451=CARTESIAN_POINT ( 'NONE',  ( 22.99824548812224378, 19.95783898428147651, 11.00732503135576401 ) ) ;
#10452=EDGE_CURVE ( 'NONE', #2599, #9431, #2976, .T. ) ;
#10459=CARTESIAN_POINT ( 'NONE',  ( -1.814555661125939912, 31.72097824480680117, 12.81469158473306713 ) ) ;
#10461=CARTESIAN_POINT ( 'NONE',  ( 23.79237391907785693, 22.55645663433636017, 11.95042449705224819 ) ) ;
#10464=CARTESIAN_POINT ( 'NONE',  ( 16.47160909572790999, 17.06392481020577279, 13.12322671172946897 ) ) ;
#10466=FILL_AREA_STYLE ('',( #10518 ) ) ;
#10479=CARTESIAN_POINT ( 'NONE',  ( -2.474873734152916338, 27.52512626584707789, 14.12500000000000355 ) ) ;
#10483=CARTESIAN_POINT ( 'NONE',  ( 0.9693646802875698354, 27.47259180932603684, 15.35718341526694530 ) ) ;
#10484=CARTESIAN_POINT ( 'NONE',  ( -1.035533905932736420, 27.49999999999998934, 14.20312500000000355 ) ) ;
#10485=CARTESIAN_POINT ( 'NONE',  ( 19.77604874367146692, 21.01153129092389094, 12.00579112326941988 ) ) ;
#10506=CARTESIAN_POINT ( 'NONE',  ( 20.78941077755876776, 23.50360388977173187, 10.95195840513859231 ) ) ;
#10512=CARTESIAN_POINT ( 'NONE',  ( 2.500000000000008438, 30.00000000000000711, 14.59375000000000178 ) ) ;
#10514=CARTESIAN_POINT ( 'NONE',  ( 23.84774077504003031, 19.42364242282459230, 10.95195840513859231 ) ) ;
#10515=CARTESIAN_POINT ( 'NONE',  ( 20.77365933115271446, 23.55783661745384094, 11.95042449705224819 ) ) ;
#10516=CARTESIAN_POINT ( 'NONE',  ( 17.17871587691444546, 17.77103159139232957, 13.12322671172946897 ) ) ;
#10518=FILL_AREA_STYLE_COLOUR ( '', #9184 ) ;
#10532=CARTESIAN_POINT ( 'NONE',  ( 1.383578242660662871, 26.47259180932604039, 16.60718341526694175 ) ) ;
#10536=CARTESIAN_POINT ( 'NONE',  ( -2.500000000000004885, 29.80321974748363090, 16.48359592357600434 ) ) ;
#10537=CARTESIAN_POINT ( 'NONE',  ( 2.500000000000008438, 30.00000000000000711, 15.84375000000000355 ) ) ;
#10538=CARTESIAN_POINT ( 'NONE',  ( 20.23853826540680600, 19.71164639310234534, 12.00579112326941988 ) ) ;
#10553=CARTESIAN_POINT ( 'NONE',  ( 19.32262643072814967, 17.24627075153934541, 11.00732576902737492 ) ) ;
#10554=EDGE_CURVE ( 'NONE', #8937, #7325, #5811, .T. ) ;
#10562=CARTESIAN_POINT ( 'NONE',  ( -2.472591809326046608, 28.89829686842208289, 14.29906658473306358 ) ) ;
#10566=CARTESIAN_POINT ( 'NONE',  ( 18.86745781575159242, 21.66267592685425569, 11.95042449705185561 ) ) ;
#10568=CARTESIAN_POINT ( 'NONE',  ( 19.12295744889739879, 19.47009535162641569, 11.95042449705107224 ) ) ;
#10569=CARTESIAN_POINT ( 'NONE',  ( 19.32345233471135515, 17.12110500680467240, 13.00476395487764947 ) ) ;
#10579=CARTESIAN_POINT ( 'NONE',  ( 22.88317621546045189, 19.71992003298075957, 12.00579112326941988 ) ) ;
#10588=CARTESIAN_POINT ( 'NONE',  ( -3.500000000000002220, 28.55025253169416288, 14.04687500000000355 ) ) ;
#10593=CARTESIAN_POINT ( 'NONE',  ( -2.479565268636987785, 29.67421718125152452, 17.49702953738633937 ) ) ;
#10594=CARTESIAN_POINT ( 'NONE',  ( 3.527408190673964494, 31.38357824266065776, 15.66968341526694175 ) ) ;
#10595=CARTESIAN_POINT ( 'NONE',  ( 22.88317621546045189, 19.71992003298075957, 12.00579112326941988 ) ) ;
#10611=CARTESIAN_POINT ( 'NONE',  ( 18.76115673388714455, 17.03897527867736983, 11.01746215567925269 ) ) ;
#10618=CARTESIAN_POINT ( 'NONE',  ( 1.767766952966372429, 31.76776695296637598, 13.50000000000000355 ) ) ;
#10622=CARTESIAN_POINT ( 'NONE',  ( 22.57450250028656669, 18.29201386669844709, 10.95195840513859231 ) ) ;
#10626=CARTESIAN_POINT ( 'NONE',  ( 20.11906803080876571, 17.66537948065741759, 13.00425721518307576 ) ) ;
#10634=CARTESIAN_POINT ( 'NONE',  ( 19.29066956973784386, 17.16581860495888634, 12.00630190750973370 ) ) ;
#10643=CARTESIAN_POINT ( 'NONE',  ( 3.500000000000007994, 29.93383077435482420, 16.84155841526694175 ) ) ;
#10647=CARTESIAN_POINT ( 'NONE',  ( 0.06616922564517249694, 32.50000000000000711, 14.65405841526694353 ) ) ;
#10662=CARTESIAN_POINT ( 'NONE',  ( 22.66010611969070965, 19.57566612754892432, 11.00732503135576401 ) ) ;
#10671=CARTESIAN_POINT ( 'NONE',  ( 24.26768760078471487, 20.42249838054411271, 10.95195840513859586 ) ) ;
#10673=CARTESIAN_POINT ( 'NONE',  ( 16.16243297953557700, 18.78731448874862053, 13.21853671947355302 ) ) ;
#10680=CARTESIAN_POINT ( 'NONE',  ( 19.69775075566884226, 17.43975236193677603, 12.00579112326941988 ) ) ;
#10686=CARTESIAN_POINT ( 'NONE',  ( 2.428085025993350410, 32.52166244231248271, 15.00219158473306535 ) ) ;
#10692=CARTESIAN_POINT ( 'NONE',  ( 1.720978244806812496, 28.18544433887406342, 15.43530841526694175 ) ) ;
#10696=CARTESIAN_POINT ( 'NONE',  ( -2.500000000000007550, 31.03553390593274131, 13.89062500000000355 ) ) ;
#10706=CARTESIAN_POINT ( 'NONE',  ( 21.41951502703731691, 22.64547864373410135, 12.00579112326941988 ) ) ;
#10714=ORIENTED_EDGE ( 'NONE', *, *, #3959, .F. ) ;
#10717=CARTESIAN_POINT ( 'NONE',  ( 20.78941077755876776, 23.50360388977173187, 10.95195840513859231 ) ) ;
#10719=CARTESIAN_POINT ( 'NONE',  ( 20.55933174294505861, 16.75535677129292722, 12.94889058896590583 ) ) ;
#10727=CARTESIAN_POINT ( 'NONE',  ( 20.23853826540680600, 19.71164639310234534, 12.00579112326941988 ) ) ;
#10735=CARTESIAN_POINT ( 'NONE',  ( -2.500000000000003997, 29.93383077435482065, 12.97094158473306358 ) ) ;
#10741=CARTESIAN_POINT ( 'NONE',  ( 0.06616922564517249694, 32.50000000000000711, 17.15405841526694175 ) ) ;
#10755=CARTESIAN_POINT ( 'NONE',  ( -3.500000000000002665, 28.55025253169416288, 14.04687500000000355 ) ) ;
#10760=CARTESIAN_POINT ( 'NONE',  ( 21.90605485701305000, 18.97586566459109392, 12.00579112326941988 ) ) ;
#10763=ORIENTED_EDGE ( 'NONE', *, *, #3083, .T. ) ;
#10765=EDGE_CURVE ( 'NONE', #2956, #5318, #10073, .T. ) ;
#10770=DIRECTION ( 'NONE',  ( -0.1561119869139967753, 0.9855205127846311530, -0.06616922564517428718 ) ) ;
#10775=CARTESIAN_POINT ( 'NONE',  ( 19.83233192245754140, 21.00689442486442360, 11.00732503135576401 ) ) ;
#10779=CARTESIAN_POINT ( 'NONE',  ( 19.49929303312607942, 16.16195407633872350, 11.95465698723049108 ) ) ;
#10786=CARTESIAN_POINT ( 'NONE',  ( 0.06616922564517314920, 33.50000000000000000, 17.15405841526694175 ) ) ;
#10790=CARTESIAN_POINT ( 'NONE',  ( 20.29953126043439227, 16.57463755921569515, 12.94889058896590583 ) ) ;
#10795=CARTESIAN_POINT ( 'NONE',  ( -0.06616922564517661864, 33.50000000000000000, 15.15844158473306535 ) ) ;
#10801=CARTESIAN_POINT ( 'NONE',  ( -2.521662442312483599, 27.57191497400664204, 15.12280841526694353 ) ) ;
#10804=CARTESIAN_POINT ( 'NONE',  ( 17.65010306112908722, 17.31038946799904465, 12.07741653513508417 ) ) ;
#10811=CARTESIAN_POINT ( 'NONE',  ( -2.474873734152920335, 32.47487373415291501, 13.81250000000000355 ) ) ;
#10817=CARTESIAN_POINT ( 'NONE',  ( 23.04535143233503192, 19.92821688535955360, 12.00579112326941988 ) ) ;
#10831=CARTESIAN_POINT ( 'NONE',  ( 15.88045857259785087, 19.06928889570832197, 12.24278471274156388 ) ) ;
#10832=( NAMED_UNIT ( * ) SI_UNIT ( $, .STERADIAN. ) SOLID_ANGLE_UNIT ( ) );
#10835=CARTESIAN_POINT ( 'NONE',  ( 18.70477062293933557, 21.09978808922912208, 12.94889058896590583 ) ) ;
#10840=CARTESIAN_POINT ( 'NONE',  ( 1.383578242660662871, 26.47259180932604039, 15.35718341526694530 ) ) ;
#10842=CARTESIAN_POINT ( 'NONE',  ( 22.92515349615029407, 19.68371071013345741, 13.00425721518307753 ) ) ;
#10847=CARTESIAN_POINT ( 'NONE',  ( 0.06616922564517943584, 27.49999999999998934, 13.28344158473306713 ) ) ;
#10848=CARTESIAN_POINT ( 'NONE',  ( 16.53922696119707325, 18.41052050710911914, 11.17880707182957600 ) ) ;
#10866=FACE_OUTER_BOUND ( 'NONE', #4056, .T. ) ;
#10870=CARTESIAN_POINT ( 'NONE',  ( 21.05771646464872404, 22.57981893131178452, 12.00579112326941988 ) ) ;
#10880=CARTESIAN_POINT ( 'NONE',  ( 17.59356678224322934, 17.35619608210146581, 12.08212522340233264 ) ) ;
#10885=CARTESIAN_POINT ( 'NONE',  ( 16.03488360227938969, 17.50065030365295016, 12.16198771834549497 ) ) ;
#10893=CARTESIAN_POINT ( 'NONE',  ( -1.383578242660661983, 33.52740819067396671, 14.73218341526694175 ) ) ;
#10895=CARTESIAN_POINT ( 'NONE',  ( 16.70557116688603472, 16.82996273904517182, 13.10128505860060066 ) ) ;
#10901=CARTESIAN_POINT ( 'NONE',  ( 2.500000000000006661, 30.06616922564517580, 13.59594158473306358 ) ) ;
#10919=PLANE ( 'NONE',  #5998 ) ;
#10928=CARTESIAN_POINT ( 'NONE',  ( 15.88045857259785087, 19.06928889570832197, 12.24278471274156388 ) ) ;
#10940=CARTESIAN_POINT ( 'NONE',  ( 18.10462311893278553, 17.05669763433401087, 12.04589798090090902 ) ) ;
#10943=CARTESIAN_POINT ( 'NONE',  ( 18.64799062861727563, 15.97503555906617123, 11.97707131907271005 ) ) ;
#10952=CARTESIAN_POINT ( 'NONE',  ( 2.474873734152918558, 32.47487373415292211, 14.75000000000000355 ) ) ;
#10956=CARTESIAN_POINT ( 'NONE',  ( 17.31044041986821469, 16.31370680995936695, 13.04945978079559765 ) ) ;
#10963=CARTESIAN_POINT ( 'NONE',  ( 1.720978244806805169, 31.81455566112594013, 15.00219158473306535 ) ) ;
#10975=CARTESIAN_POINT ( 'NONE',  ( 23.33980466280999977, 20.94445964013513617, 12.00579112326902909 ) ) ;
ENDSEC;
END-ISO-10303-21;
